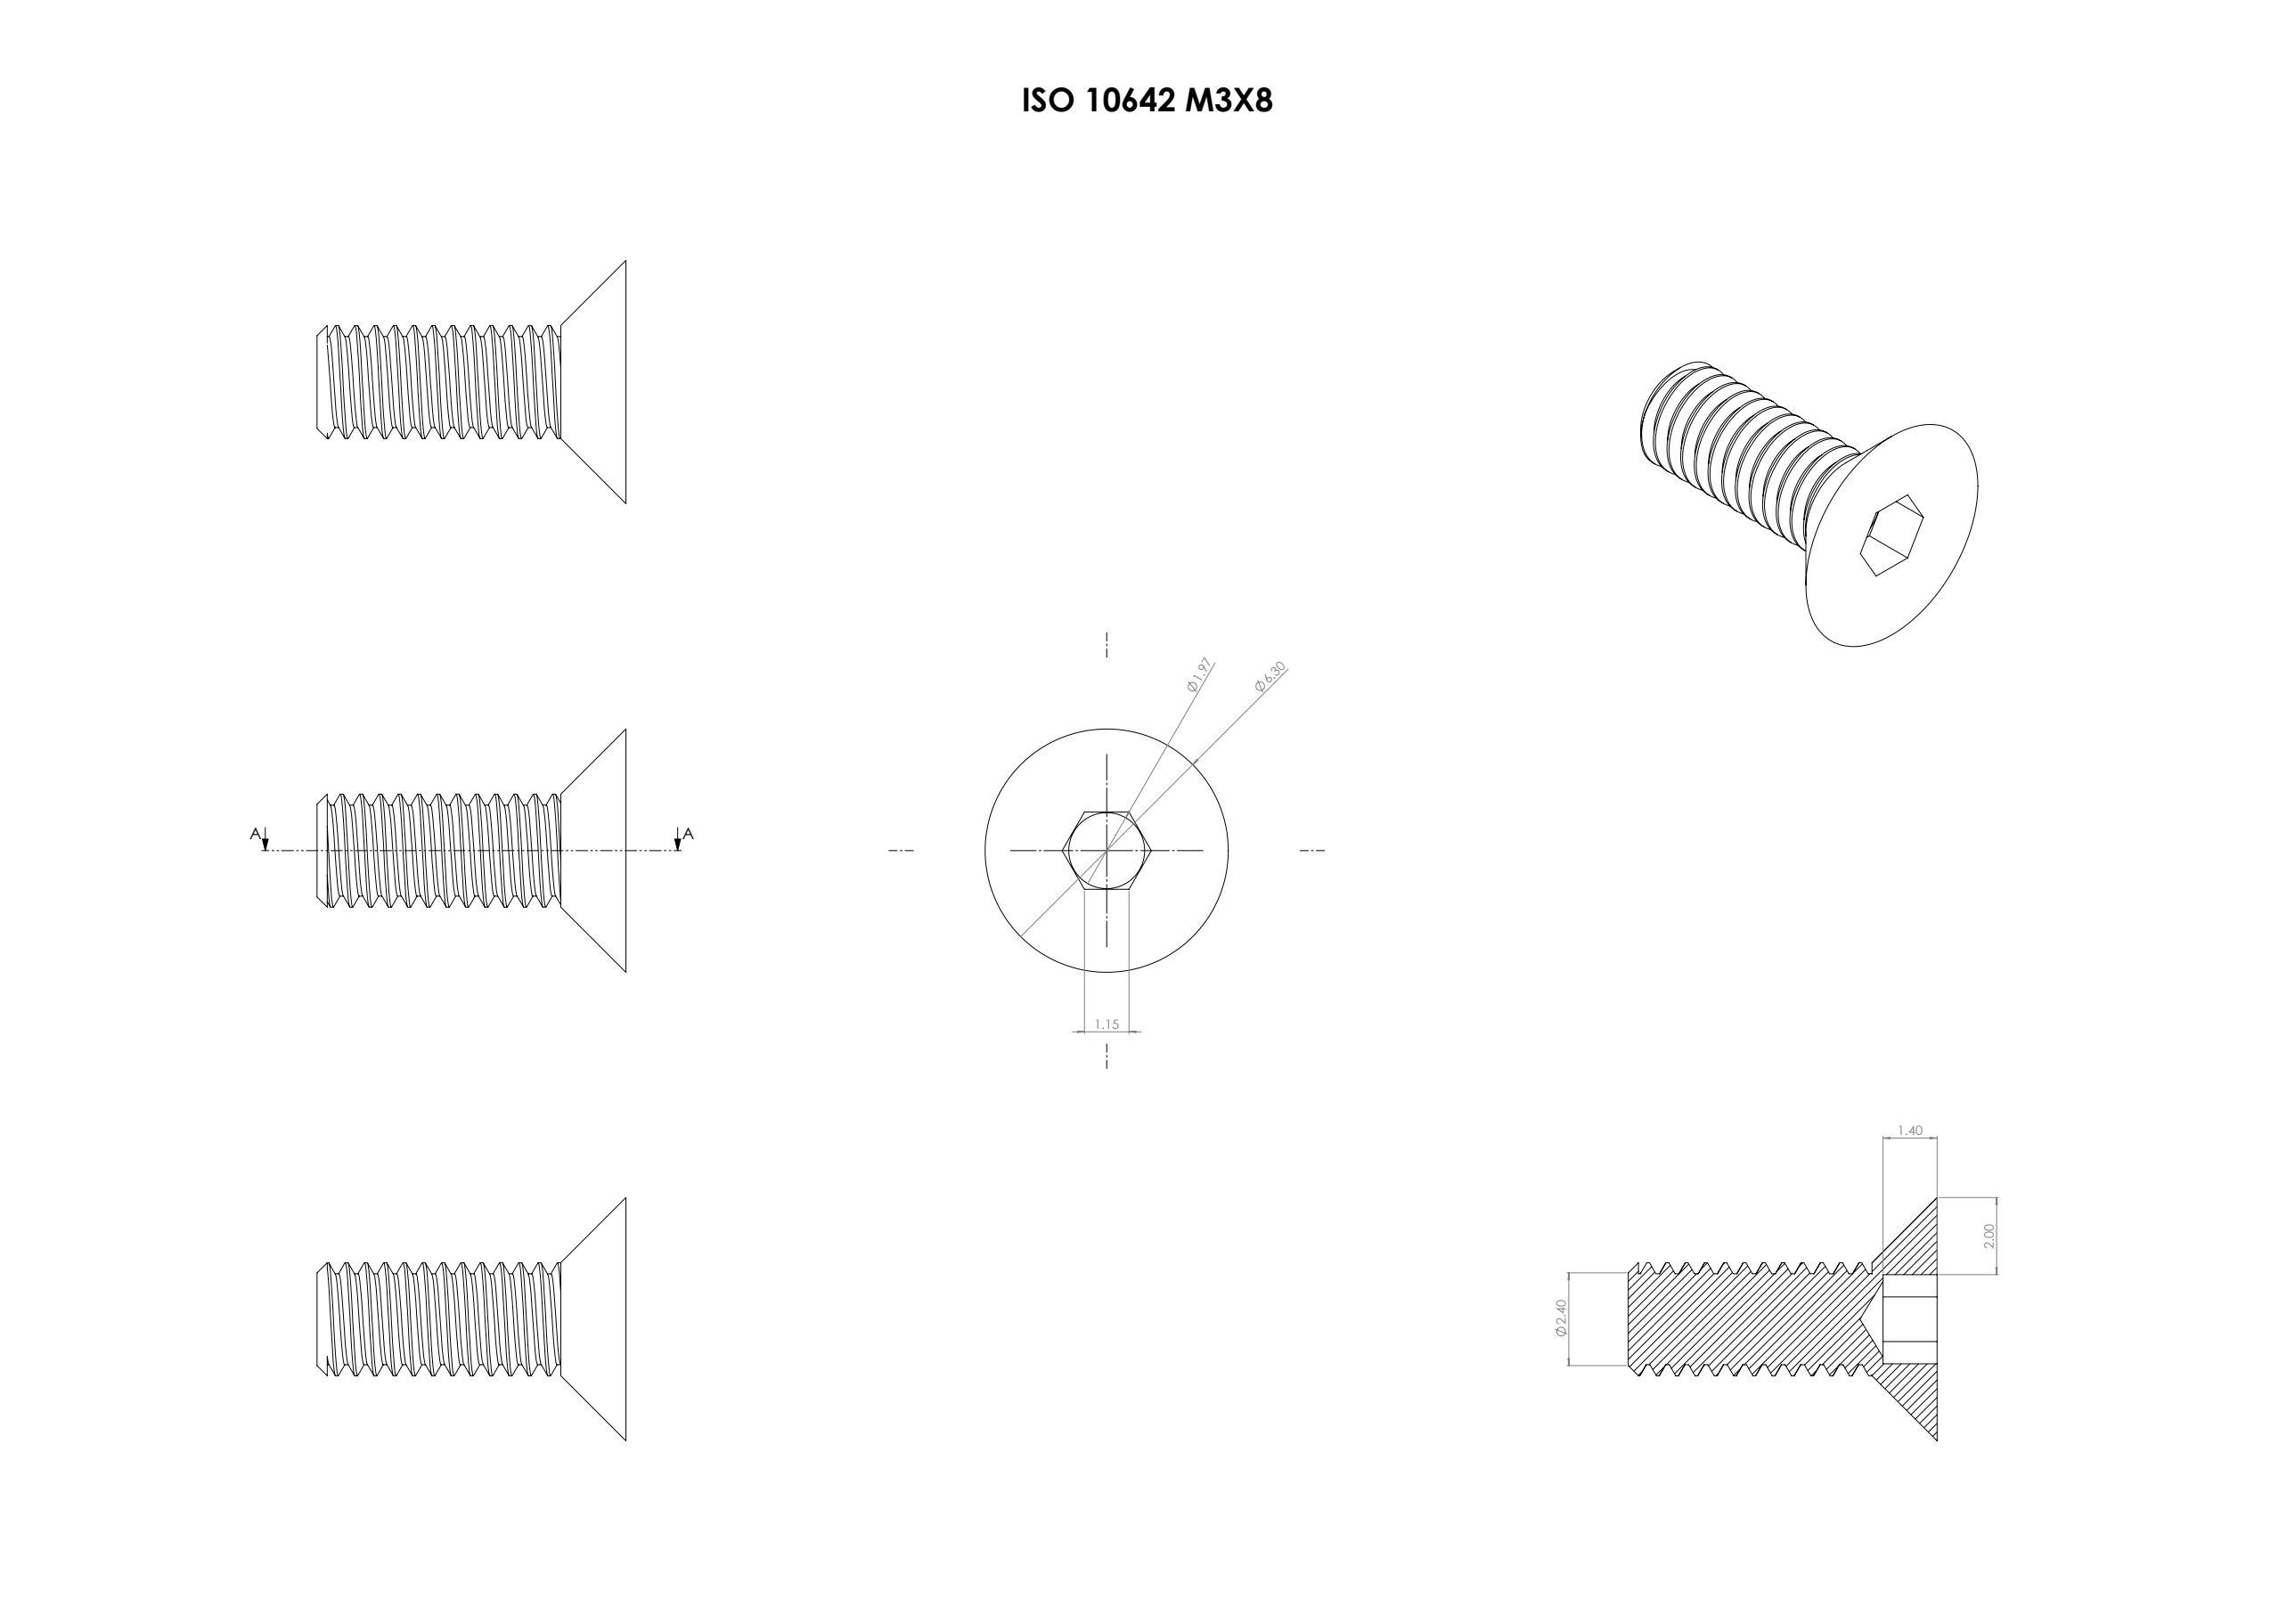
ISO-10303-21;
HEADER;
/* Generated by software containing ST-Developer
 * from STEP Tools, Inc. (www.steptools.com) 
 */

FILE_DESCRIPTION(
/* description */ (''),
/* implementation_level */ '2;1');

FILE_NAME(
/* name */ '11_ISO_10642_M3x8.step',
/* time_stamp */ '2026-10-21T01:59:45-07:00',
/* author */ (''),
/* organization */ (''),
/* preprocessor_version */ 'ST-DEVELOPER v20.2',
/* originating_system */ 'Autodesk Translation Framework v15.15.0.0',
/* authorisation */ '');

FILE_SCHEMA (('AUTOMOTIVE_DESIGN { 1 0 10303 214 3 1 1 }'));
ENDSEC;

DATA;
#10=MECHANICAL_DESIGN_GEOMETRIC_PRESENTATION_REPRESENTATION('',(#479),#18281);
#186=B_SPLINE_SURFACE_WITH_KNOTS('',3,3,((#17274,#17275,#17276,#17277,#17278,
#17279,#17280,#17281,#17282,#17283,#17284,#17285,#17286,#17287,#17288,#17289,
#17290,#17291,#17292,#17293,#17294,#17295,#17296,#17297,#17298,#17299,#17300,
#17301,#17302,#17303,#17304,#17305,#17306,#17307,#17308,#17309,#17310,#17311,
#17312,#17313,#17314,#17315,#17316,#17317,#17318,#17319,#17320,#17321,#17322,
#17323,#17324,#17325,#17326,#17327,#17328,#17329,#17330,#17331,#17332,#17333,
#17334,#17335,#17336,#17337,#17338,#17339,#17340,#17341,#17342,#17343,#17344,
#17345,#17346,#17347,#17348,#17349,#17350,#17351,#17352,#17353,#17354,#17355),
(#17356,#17357,#17358,#17359,#17360,#17361,#17362,#17363,#17364,#17365,
#17366,#17367,#17368,#17369,#17370,#17371,#17372,#17373,#17374,#17375,#17376,
#17377,#17378,#17379,#17380,#17381,#17382,#17383,#17384,#17385,#17386,#17387,
#17388,#17389,#17390,#17391,#17392,#17393,#17394,#17395,#17396,#17397,#17398,
#17399,#17400,#17401,#17402,#17403,#17404,#17405,#17406,#17407,#17408,#17409,
#17410,#17411,#17412,#17413,#17414,#17415,#17416,#17417,#17418,#17419,#17420,
#17421,#17422,#17423,#17424,#17425,#17426,#17427,#17428,#17429,#17430,#17431,
#17432,#17433,#17434,#17435,#17436,#17437),(#17438,#17439,#17440,#17441,
#17442,#17443,#17444,#17445,#17446,#17447,#17448,#17449,#17450,#17451,#17452,
#17453,#17454,#17455,#17456,#17457,#17458,#17459,#17460,#17461,#17462,#17463,
#17464,#17465,#17466,#17467,#17468,#17469,#17470,#17471,#17472,#17473,#17474,
#17475,#17476,#17477,#17478,#17479,#17480,#17481,#17482,#17483,#17484,#17485,
#17486,#17487,#17488,#17489,#17490,#17491,#17492,#17493,#17494,#17495,#17496,
#17497,#17498,#17499,#17500,#17501,#17502,#17503,#17504,#17505,#17506,#17507,
#17508,#17509,#17510,#17511,#17512,#17513,#17514,#17515,#17516,#17517,#17518,
#17519),(#17520,#17521,#17522,#17523,#17524,#17525,#17526,#17527,#17528,
#17529,#17530,#17531,#17532,#17533,#17534,#17535,#17536,#17537,#17538,#17539,
#17540,#17541,#17542,#17543,#17544,#17545,#17546,#17547,#17548,#17549,#17550,
#17551,#17552,#17553,#17554,#17555,#17556,#17557,#17558,#17559,#17560,#17561,
#17562,#17563,#17564,#17565,#17566,#17567,#17568,#17569,#17570,#17571,#17572,
#17573,#17574,#17575,#17576,#17577,#17578,#17579,#17580,#17581,#17582,#17583,
#17584,#17585,#17586,#17587,#17588,#17589,#17590,#17591,#17592,#17593,#17594,
#17595,#17596,#17597,#17598,#17599,#17600,#17601)),.UNSPECIFIED.,.F.,.F.,
 .F.,(4,4),(4,1,1,1,1,1,1,1,1,1,1,1,1,1,1,1,1,1,1,1,1,1,1,1,1,1,1,1,1,1,
1,1,1,1,1,1,1,1,1,1,1,1,1,1,1,1,1,1,1,1,1,1,1,1,1,1,1,1,1,1,1,1,1,1,1,1,
1,1,1,1,1,1,1,1,1,1,1,1,1,4),(0.,0.0329955678841871),(8.30203615430834,
9.29064014026014,10.2792441262119,11.2678481121638,12.2564520981156,13.2450560840674,
14.2336600700192,15.222264055971,16.2108680419228,17.1994720278746,18.1880760138264,
19.1766799997782,20.16528398573,21.1538879716818,22.1424919576336,23.1310959435854,
24.1196999295372,25.108303915489,26.0969079014409,27.0855118873927,28.0741158733445,
29.0627198592963,30.0513238452481,31.0399278311999,32.0285318171517,33.0171358031035,
34.0057397890553,34.9943437750071,35.9829477609589,36.9715517469107,37.9601557328625,
38.9487597188143,39.9373637047661,40.9259676907179,41.9145716766698,42.9031756626216,
43.8917796485734,44.8803836345252,45.868987620477,46.8575916064288,47.8461955923806,
48.8347995783324,49.8234035642842,50.812007550236,51.8006115361878,52.7892155221396,
53.7778195080914,54.7664234940432,55.755027479995,56.7436314659468,57.7322354518986,
58.7208394378505,59.7094434238023,60.6980474097541,61.6866513957059,62.6752553816577,
63.6638593676095,64.6524633535613,65.6410673395131,66.6296713254649,67.6182753114167,
68.6068792973685,69.5954832833203,70.5840872692721,71.5726912552239,72.5612952411758,
73.5498992271276,74.5385032130794,75.5271071990312,76.515711184983,77.5043151709348,
78.4929191568866,79.4815231428384,80.4701271287902,81.458731114742,82.4473351006938,
83.4359390866456,84.4245430725974,85.4131470585492,86.401751044501),
 .UNSPECIFIED.);
#187=B_SPLINE_SURFACE_WITH_KNOTS('',3,3,((#17813,#17814,#17815,#17816,#17817,
#17818,#17819,#17820,#17821,#17822,#17823,#17824,#17825,#17826,#17827,#17828,
#17829,#17830,#17831,#17832,#17833,#17834,#17835,#17836,#17837,#17838,#17839,
#17840,#17841,#17842,#17843,#17844,#17845,#17846,#17847,#17848,#17849,#17850,
#17851,#17852,#17853,#17854,#17855,#17856,#17857,#17858,#17859,#17860,#17861,
#17862,#17863,#17864,#17865,#17866,#17867,#17868,#17869,#17870,#17871,#17872,
#17873,#17874,#17875,#17876,#17877,#17878,#17879,#17880,#17881,#17882,#17883,
#17884,#17885,#17886,#17887,#17888,#17889,#17890,#17891,#17892,#17893,#17894),
(#17895,#17896,#17897,#17898,#17899,#17900,#17901,#17902,#17903,#17904,
#17905,#17906,#17907,#17908,#17909,#17910,#17911,#17912,#17913,#17914,#17915,
#17916,#17917,#17918,#17919,#17920,#17921,#17922,#17923,#17924,#17925,#17926,
#17927,#17928,#17929,#17930,#17931,#17932,#17933,#17934,#17935,#17936,#17937,
#17938,#17939,#17940,#17941,#17942,#17943,#17944,#17945,#17946,#17947,#17948,
#17949,#17950,#17951,#17952,#17953,#17954,#17955,#17956,#17957,#17958,#17959,
#17960,#17961,#17962,#17963,#17964,#17965,#17966,#17967,#17968,#17969,#17970,
#17971,#17972,#17973,#17974,#17975,#17976),(#17977,#17978,#17979,#17980,
#17981,#17982,#17983,#17984,#17985,#17986,#17987,#17988,#17989,#17990,#17991,
#17992,#17993,#17994,#17995,#17996,#17997,#17998,#17999,#18000,#18001,#18002,
#18003,#18004,#18005,#18006,#18007,#18008,#18009,#18010,#18011,#18012,#18013,
#18014,#18015,#18016,#18017,#18018,#18019,#18020,#18021,#18022,#18023,#18024,
#18025,#18026,#18027,#18028,#18029,#18030,#18031,#18032,#18033,#18034,#18035,
#18036,#18037,#18038,#18039,#18040,#18041,#18042,#18043,#18044,#18045,#18046,
#18047,#18048,#18049,#18050,#18051,#18052,#18053,#18054,#18055,#18056,#18057,
#18058),(#18059,#18060,#18061,#18062,#18063,#18064,#18065,#18066,#18067,
#18068,#18069,#18070,#18071,#18072,#18073,#18074,#18075,#18076,#18077,#18078,
#18079,#18080,#18081,#18082,#18083,#18084,#18085,#18086,#18087,#18088,#18089,
#18090,#18091,#18092,#18093,#18094,#18095,#18096,#18097,#18098,#18099,#18100,
#18101,#18102,#18103,#18104,#18105,#18106,#18107,#18108,#18109,#18110,#18111,
#18112,#18113,#18114,#18115,#18116,#18117,#18118,#18119,#18120,#18121,#18122,
#18123,#18124,#18125,#18126,#18127,#18128,#18129,#18130,#18131,#18132,#18133,
#18134,#18135,#18136,#18137,#18138,#18139,#18140)),.UNSPECIFIED.,.F.,.F.,
 .F.,(4,4),(4,1,1,1,1,1,1,1,1,1,1,1,1,1,1,1,1,1,1,1,1,1,1,1,1,1,1,1,1,1,
1,1,1,1,1,1,1,1,1,1,1,1,1,1,1,1,1,1,1,1,1,1,1,1,1,1,1,1,1,1,1,1,1,1,1,1,
1,1,1,1,1,1,1,1,1,1,1,1,1,4),(0.,0.0329955678841871),(11.6159397475004,
12.6045437334522,13.593147719404,14.5817517053558,15.5703556913076,16.5589596772594,
17.5475636632112,18.536167649163,19.5247716351148,20.5133756210666,21.5019796070184,
22.4905835929702,23.479187578922,24.4677915648739,25.4563955508257,26.4449995367775,
27.4336035227293,28.4222075086811,29.4108114946329,30.3994154805847,31.3880194665365,
32.3766234524883,33.3652274384401,34.3538314243919,35.3424354103437,36.3310393962955,
37.3196433822473,38.3082473681991,39.296851354151,40.2854553401028,41.2740593260546,
42.2626633120064,43.2512672979582,44.23987128391,45.2284752698618,46.2170792558136,
47.2056832417654,48.1942872277172,49.182891213669,50.1714951996208,51.1600991855726,
52.1487031715244,53.1373071574762,54.1259111434281,55.1145151293799,56.1031191153317,
57.0917231012835,58.0803270872353,59.0689310731871,60.0575350591389,61.0461390450907,
62.0347430310425,63.0233470169943,64.0119510029461,65.0005549888979,65.9891589748497,
66.9777629608015,67.9663669467533,68.9549709327052,69.943574918657,70.9321789046088,
71.9207828905606,72.9093868765124,73.8979908624642,74.886594848416,75.8751988343678,
76.8638028203196,77.8524068062714,78.8410107922232,79.829614778175,80.8182187641268,
81.8068227500786,82.7954267360304,83.7840307219822,84.7726347079341,85.7612386938859,
86.7498426798377,87.7384466657895,88.7270506517413,89.7156546376931),
 .UNSPECIFIED.);
#312=B_SPLINE_CURVE_WITH_KNOTS('',3,(#16240,#16241,#16242,#16243,#16244,
#16245,#16246,#16247,#16248,#16249),.UNSPECIFIED.,.F.,.F.,(4,3,3,4),(-4.09202352044854,
-3.95441594380723,-2.96581195785542,-2.07317267331972),.UNSPECIFIED.);
#313=B_SPLINE_CURVE_WITH_KNOTS('',3,(#16252,#16253,#16254,#16255,#16256,
#16257,#16258),.UNSPECIFIED.,.F.,.F.,(4,3,4),(0.,0.98860398595181,1.12274180646091),
 .UNSPECIFIED.);
#314=B_SPLINE_CURVE_WITH_KNOTS('',3,(#16263,#16264,#16265,#16266,#16267,
#16268,#16269,#16270,#16271,#16272,#16273,#16274,#16275,#16276,#16277,#16278,
#16279,#16280,#16281,#16282,#16283,#16284),.UNSPECIFIED.,.F.,.F.,(4,3,3,
3,3,3,3,4),(-10.3752088276281,-9.88603985951807,-8.89743587356626,-7.90883188761445,
-6.92022790166265,-5.93162391571084,-4.94301992975903,-4.09202352044854),
 .UNSPECIFIED.);
#315=B_SPLINE_CURVE_WITH_KNOTS('',3,(#16285,#16286,#16287,#16288,#16289,
#16290,#16291,#16292,#16293,#16294,#16295,#16296,#16297,#16298,#16299,#16300,
#16301,#16302,#16303,#16304,#16305,#16306),.UNSPECIFIED.,.F.,.F.,(4,3,3,
3,3,3,3,4),(1.12274180646091,1.97720797190362,2.96581195785542,3.95441594380723,
4.94301992975904,5.93162391571084,6.92022790166265,7.4059271136405),
 .UNSPECIFIED.);
#316=B_SPLINE_CURVE_WITH_KNOTS('',3,(#16311,#16312,#16313,#16314,#16315,
#16316,#16317,#16318,#16319,#16320,#16321,#16322,#16323,#16324,#16325,#16326,
#16327,#16328,#16329,#16330,#16331,#16332),.UNSPECIFIED.,.F.,.F.,(4,3,3,
3,3,3,3,4),(-16.6583941348077,-15.8176637752289,-14.8290597892771,-13.8404558033253,
-12.8518518173735,-11.8632478314217,-10.8746438454699,-10.3752088276281),
 .UNSPECIFIED.);
#317=B_SPLINE_CURVE_WITH_KNOTS('',3,(#16333,#16334,#16335,#16336,#16337,
#16338,#16339,#16340,#16341,#16342,#16343,#16344,#16345,#16346,#16347,#16348,
#16349,#16350,#16351,#16352,#16353,#16354),.UNSPECIFIED.,.F.,.F.,(4,3,3,
3,3,3,3,4),(7.4059271136405,7.90883188761445,8.89743587356626,9.88603985951806,
10.8746438454699,11.8632478314217,12.8518518173735,13.6891124208201),
 .UNSPECIFIED.);
#318=B_SPLINE_CURVE_WITH_KNOTS('',3,(#16359,#16360,#16361,#16362,#16363,
#16364,#16365,#16366,#16367,#16368,#16369,#16370,#16371,#16372,#16373,#16374,
#16375,#16376,#16377,#16378,#16379,#16380,#16381,#16382,#16383),
 .UNSPECIFIED.,.F.,.F.,(4,3,3,3,3,3,3,3,4),(-22.9415794419873,-22.7378916768916,
-21.7492876909397,-20.7606837049879,-19.7720797190361,-18.7834757330843,
-17.7948717471325,-16.8062677611807,-16.6583941348077),.UNSPECIFIED.);
#319=B_SPLINE_CURVE_WITH_KNOTS('',3,(#16384,#16385,#16386,#16387,#16388,
#16389,#16390,#16391,#16392,#16393,#16394,#16395,#16396,#16397,#16398,#16399,
#16400,#16401,#16402,#16403,#16404,#16405,#16406,#16407,#16408),
 .UNSPECIFIED.,.F.,.F.,(4,3,3,3,3,3,3,3,4),(13.6891124208201,13.8404558033253,
14.8290597892771,15.8176637752289,16.8062677611807,17.7948717471325,18.7834757330843,
19.7720797190361,19.9722977279997),.UNSPECIFIED.);
#320=B_SPLINE_CURVE_WITH_KNOTS('',3,(#16413,#16414,#16415,#16416,#16417,
#16418,#16419,#16420,#16421,#16422,#16423,#16424,#16425,#16426,#16427,#16428,
#16429,#16430,#16431,#16432,#16433,#16434),.UNSPECIFIED.,.F.,.F.,(4,3,3,
3,3,3,3,4),(-29.2247647491669,-28.6695155926024,-27.6809116066506,-26.6923076206988,
-25.703703634747,-24.7150996487952,-23.7264956628434,-22.9415794419873),
 .UNSPECIFIED.);
#321=B_SPLINE_CURVE_WITH_KNOTS('',3,(#16435,#16436,#16437,#16438,#16439,
#16440,#16441,#16442,#16443,#16444,#16445,#16446,#16447,#16448,#16449,#16450,
#16451,#16452,#16453,#16454,#16455,#16456),.UNSPECIFIED.,.F.,.F.,(4,3,3,
3,3,3,3,4),(19.9722977279997,20.7606837049879,21.7492876909397,22.7378916768916,
23.7264956628434,24.7150996487952,25.703703634747,26.2554830351793),
 .UNSPECIFIED.);
#322=B_SPLINE_CURVE_WITH_KNOTS('',3,(#16461,#16462,#16463,#16464,#16465,
#16466,#16467,#16468,#16469,#16470,#16471,#16472,#16473,#16474,#16475,#16476,
#16477,#16478,#16479,#16480,#16481,#16482),.UNSPECIFIED.,.F.,.F.,(4,3,3,
3,3,3,3,4),(-35.5079500563465,-34.6011395083132,-33.6125355223614,-32.6239315364096,
-31.6353275504578,-30.646723564506,-29.6581195785542,-29.2247647491669),
 .UNSPECIFIED.);
#323=B_SPLINE_CURVE_WITH_KNOTS('',3,(#16483,#16484,#16485,#16486,#16487,
#16488,#16489,#16490,#16491,#16492,#16493,#16494,#16495,#16496,#16497,#16498,
#16499,#16500,#16501,#16502,#16503,#16504),.UNSPECIFIED.,.F.,.F.,(4,3,3,
3,3,3,3,4),(26.2554830351793,26.6923076206988,27.6809116066506,28.6695155926024,
29.6581195785542,30.646723564506,31.6353275504578,32.5386683423588),
 .UNSPECIFIED.);
#324=B_SPLINE_CURVE_WITH_KNOTS('',3,(#16509,#16510,#16511,#16512,#16513,
#16514,#16515,#16516,#16517,#16518,#16519,#16520,#16521,#16522,#16523,#16524,
#16525,#16526,#16527,#16528,#16529,#16530,#16531,#16532,#16533),
 .UNSPECIFIED.,.F.,.F.,(4,3,3,3,3,3,3,3,4),(-41.7911353635261,-41.5213674099759,
-40.5327634240241,-39.5441594380723,-38.5555554521205,-37.5669514661687,
-36.5783474802168,-35.589743494265,-35.5079500563465),.UNSPECIFIED.);
#325=B_SPLINE_CURVE_WITH_KNOTS('',3,(#16534,#16535,#16536,#16537,#16538,
#16539,#16540,#16541,#16542,#16543,#16544,#16545,#16546,#16547,#16548,#16549,
#16550,#16551,#16552,#16553,#16554,#16555,#16556,#16557,#16558),
 .UNSPECIFIED.,.F.,.F.,(4,3,3,3,3,3,3,3,4),(32.5386683423588,32.6239315364096,
33.6125355223614,34.6011395083132,35.589743494265,36.5783474802168,37.5669514661686,
38.5555554521205,38.8218536495384),.UNSPECIFIED.);
#326=B_SPLINE_CURVE_WITH_KNOTS('',3,(#16563,#16564,#16565,#16566,#16567,
#16568,#16569,#16570,#16571,#16572,#16573,#16574,#16575,#16576,#16577,#16578,
#16579,#16580,#16581,#16582,#16583,#16584),.UNSPECIFIED.,.F.,.F.,(4,3,3,
3,3,3,3,4),(-48.0743206707057,-47.4529913256867,-46.4643873397349,-45.4757833537831,
-44.4871793678313,-43.4985753818795,-42.5099713959277,-41.7911353635261),
 .UNSPECIFIED.);
#327=B_SPLINE_CURVE_WITH_KNOTS('',3,(#16585,#16586,#16587,#16588,#16589,
#16590,#16591,#16592,#16593,#16594,#16595,#16596,#16597,#16598,#16599,#16600,
#16601,#16602,#16603,#16604,#16605,#16606),.UNSPECIFIED.,.F.,.F.,(4,3,3,
3,3,3,3,4),(38.8218536495384,39.5441594380723,40.5327634240241,41.5213674099759,
42.5099713959277,43.4985753818795,44.4871793678313,45.105038956718),
 .UNSPECIFIED.);
#328=B_SPLINE_CURVE_WITH_KNOTS('',3,(#16611,#16612,#16613,#16614,#16615,
#16616,#16617,#16618,#16619,#16620,#16621,#16622,#16623,#16624,#16625,#16626,
#16627,#16628,#16629,#16630,#16631,#16632),.UNSPECIFIED.,.F.,.F.,(4,3,3,
3,3,3,3,4),(-54.3575059778853,-53.3846152413976,-52.3960112554458,-51.4074072694939,
-50.4188032835421,-49.4301992975903,-48.4415953116385,-48.0743206707057),
 .UNSPECIFIED.);
#329=B_SPLINE_CURVE_WITH_KNOTS('',3,(#16633,#16634,#16635,#16636,#16637,
#16638,#16639,#16640,#16641,#16642,#16643,#16644,#16645,#16646,#16647,#16648,
#16649,#16650,#16651,#16652,#16653,#16654),.UNSPECIFIED.,.F.,.F.,(4,3,3,
3,3,3,3,4),(45.105038956718,45.4757833537831,46.4643873397349,47.4529913256867,
48.4415953116385,49.4301992975903,50.4188032835421,51.3882242638976),
 .UNSPECIFIED.);
#330=B_SPLINE_CURVE_WITH_KNOTS('',3,(#16659,#16660,#16661,#16662,#16663,
#16664,#16665,#16666,#16667,#16668,#16669,#16670,#16671,#16672,#16673,#16674,
#16675,#16676,#16677,#16678,#16679,#16680,#16681,#16682,#16683),
 .UNSPECIFIED.,.F.,.F.,(4,3,3,3,3,3,3,3,4),(-60.6406912850648,-60.3048431430602,
-59.3162391571084,-58.3276351711566,-57.3390311852048,-56.350427199253,
-55.3618232133012,-54.3732192273494,-54.3575059778853),.UNSPECIFIED.);
#331=B_SPLINE_CURVE_WITH_KNOTS('',3,(#16684,#16685,#16686,#16687,#16688,
#16689,#16690,#16691,#16692,#16693,#16694,#16695,#16696,#16697,#16698,#16699,
#16700,#16701,#16702,#16703,#16704,#16705,#16706,#16707,#16708),
 .UNSPECIFIED.,.F.,.F.,(4,3,3,3,3,3,3,3,4),(51.3882242638976,51.4074072694939,
52.3960112554457,53.3846152413976,54.3732192273494,55.3618232133012,56.350427199253,
57.3390311852048,57.6714095710772),.UNSPECIFIED.);
#332=B_SPLINE_CURVE_WITH_KNOTS('',3,(#16713,#16714,#16715,#16716,#16717,
#16718,#16719,#16720,#16721,#16722,#16723,#16724,#16725,#16726,#16727,#16728,
#16729,#16730,#16731,#16732,#16733,#16734),.UNSPECIFIED.,.F.,.F.,(4,3,3,
3,3,3,3,4),(-66.9238765922444,-66.236467058771,-65.2478630728192,-64.2592590868674,
-63.2706551009156,-62.2820511149638,-61.293447129012,-60.6406912850648),
 .UNSPECIFIED.);
#333=B_SPLINE_CURVE_WITH_KNOTS('',3,(#16735,#16736,#16737,#16738,#16739,
#16740,#16741,#16742,#16743,#16744,#16745,#16746,#16747,#16748,#16749,#16750,
#16751,#16752,#16753,#16754,#16755,#16756),.UNSPECIFIED.,.F.,.F.,(4,3,3,
3,3,3,3,4),(57.6714095710772,58.3276351711566,59.3162391571084,60.3048431430602,
61.293447129012,62.2820511149638,63.2706551009156,63.9545948782568),
 .UNSPECIFIED.);
#334=B_SPLINE_CURVE_WITH_KNOTS('',3,(#16761,#16762,#16763,#16764,#16765,
#16766,#16767,#16768,#16769,#16770,#16771,#16772,#16773,#16774,#16775,#16776,
#16777,#16778,#16779,#16780,#16781,#16782,#16783,#16784,#16785),
 .UNSPECIFIED.,.F.,.F.,(4,3,3,3,3,3,3,3,4),(-73.207061899424,-73.1566949604337,
-72.1680909744819,-71.1794869885301,-70.1908830025783,-69.2022790166264,
-68.2136750306747,-67.2250710447229,-66.9238765922444),.UNSPECIFIED.);
#335=B_SPLINE_CURVE_WITH_KNOTS('',3,(#16786,#16787,#16788,#16789,#16790,
#16791,#16792,#16793,#16794,#16795,#16796,#16797,#16798,#16799,#16800,#16801,
#16802,#16803,#16804,#16805,#16806,#16807,#16808,#16809,#16810),
 .UNSPECIFIED.,.F.,.F.,(4,3,3,3,3,3,3,3,4),(63.9545948782568,64.2592590868674,
65.2478630728192,66.236467058771,67.2250710447228,68.2136750306746,69.2022790166264,
70.1908830025782,70.2377801854364),.UNSPECIFIED.);
#336=B_SPLINE_CURVE_WITH_KNOTS('',3,(#16816,#16817,#16818,#16819,#16820,
#16821),.UNSPECIFIED.,.F.,.F.,(4,1,1,4),(84.8230016469244,85.7612386938859,
86.7498426798377,87.6424819643734),.UNSPECIFIED.);
#337=B_SPLINE_CURVE_WITH_KNOTS('',3,(#16824,#16825,#16826,#16827,#16828),
 .UNSPECIFIED.,.F.,.F.,(4,1,4),(84.8230016469244,85.4131470585492,86.401751044501),
 .UNSPECIFIED.);
#338=B_SPLINE_CURVE_WITH_KNOTS('',3,(#16833,#16834,#16835,#16836,#16837,
#16838,#16839,#16840,#16841,#16842,#16843),.UNSPECIFIED.,.F.,.F.,(4,1,1,
1,1,1,1,1,4),(78.5398163397448,78.8410107922232,79.829614778175,80.8182187641268,
81.8068227500786,82.7954267360304,83.7840307219822,84.7726347079341,84.8230016469244),
 .UNSPECIFIED.);
#339=B_SPLINE_CURVE_WITH_KNOTS('',3,(#16844,#16845,#16846,#16847,#16848,
#16849,#16850,#16851,#16852,#16853),.UNSPECIFIED.,.F.,.F.,(4,1,1,1,1,1,
1,4),(78.5398163397448,79.4815231428384,80.4701271287902,81.458731114742,
82.4473351006938,83.4359390866456,84.4245430725974,84.8230016469244),
 .UNSPECIFIED.);
#340=B_SPLINE_CURVE_WITH_KNOTS('',3,(#16858,#16859,#16860,#16861,#16862,
#16863,#16864,#16865,#16866,#16867),.UNSPECIFIED.,.F.,.F.,(4,1,1,1,1,1,
1,4),(72.2566310325652,72.9093868765124,73.8979908624642,74.886594848416,
75.8751988343678,76.8638028203196,77.8524068062714,78.5398163397448),
 .UNSPECIFIED.);
#341=B_SPLINE_CURVE_WITH_KNOTS('',3,(#16868,#16869,#16870,#16871,#16872,
#16873,#16874,#16875,#16876,#16877,#16878),.UNSPECIFIED.,.F.,.F.,(4,1,1,
1,1,1,1,1,4),(72.2566310325652,72.5612952411758,73.5498992271276,74.5385032130794,
75.5271071990312,76.515711184983,77.5043151709348,78.4929191568866,78.5398163397448),
 .UNSPECIFIED.);
#342=B_SPLINE_CURVE_WITH_KNOTS('',3,(#16883,#16884,#16885,#16886,#16887,
#16888,#16889,#16890,#16891,#16892,#16893),.UNSPECIFIED.,.F.,.F.,(4,1,1,
1,1,1,1,1,4),(65.9734457253856,65.9891589748497,66.9777629608015,67.9663669467533,
68.9549709327052,69.943574918657,70.9321789046088,71.9207828905606,72.2566310325652),
 .UNSPECIFIED.);
#343=B_SPLINE_CURVE_WITH_KNOTS('',3,(#16894,#16895,#16896,#16897,#16898,
#16899,#16900,#16901,#16902,#16903),.UNSPECIFIED.,.F.,.F.,(4,1,1,1,1,1,
1,4),(65.9734457253856,66.6296713254649,67.6182753114167,68.6068792973685,
69.5954832833203,70.5840872692721,71.5726912552239,72.2566310325652),
 .UNSPECIFIED.);
#344=B_SPLINE_CURVE_WITH_KNOTS('',3,(#16908,#16909,#16910,#16911,#16912,
#16913,#16914,#16915,#16916,#16917),.UNSPECIFIED.,.F.,.F.,(4,1,1,1,1,1,
1,4),(59.6902604182061,60.0575350591389,61.0461390450907,62.0347430310425,
63.0233470169943,64.0119510029461,65.0005549888979,65.9734457253856),
 .UNSPECIFIED.);
#345=B_SPLINE_CURVE_WITH_KNOTS('',3,(#16918,#16919,#16920,#16921,#16922,
#16923,#16924,#16925,#16926,#16927,#16928),.UNSPECIFIED.,.F.,.F.,(4,1,1,
1,1,1,1,1,4),(59.690260418206,59.7094434238023,60.6980474097541,61.6866513957059,
62.6752553816577,63.6638593676095,64.6524633535613,65.6410673395131,65.9734457253856),
 .UNSPECIFIED.);
#346=B_SPLINE_CURVE_WITH_KNOTS('',3,(#16933,#16934,#16935,#16936,#16937,
#16938,#16939,#16940,#16941,#16942),.UNSPECIFIED.,.F.,.F.,(4,1,1,1,1,1,
1,4),(53.4070751110265,54.1259111434281,55.1145151293799,56.1031191153317,
57.0917231012835,58.0803270872353,59.0689310731871,59.6902604182061),
 .UNSPECIFIED.);
#347=B_SPLINE_CURVE_WITH_KNOTS('',3,(#16943,#16944,#16945,#16946,#16947,
#16948,#16949,#16950,#16951,#16952),.UNSPECIFIED.,.F.,.F.,(4,1,1,1,1,1,
1,4),(53.4070751110264,53.7778195080914,54.7664234940432,55.755027479995,
56.7436314659468,57.7322354518986,58.7208394378505,59.690260418206),
 .UNSPECIFIED.);
#348=B_SPLINE_CURVE_WITH_KNOTS('',3,(#16957,#16958,#16959,#16960,#16961,
#16962,#16963,#16964,#16965,#16966,#16967),.UNSPECIFIED.,.F.,.F.,(4,1,1,
1,1,1,1,1,4),(47.1238898038469,47.2056832417654,48.1942872277172,49.182891213669,
50.1714951996208,51.1600991855726,52.1487031715244,53.1373071574762,53.4070751110265),
 .UNSPECIFIED.);
#349=B_SPLINE_CURVE_WITH_KNOTS('',3,(#16968,#16969,#16970,#16971,#16972,
#16973,#16974,#16975,#16976,#16977),.UNSPECIFIED.,.F.,.F.,(4,1,1,1,1,1,
1,4),(47.1238898038468,47.8461955923806,48.8347995783324,49.8234035642842,
50.812007550236,51.8006115361878,52.7892155221396,53.4070751110264),
 .UNSPECIFIED.);
#350=B_SPLINE_CURVE_WITH_KNOTS('',3,(#16982,#16983,#16984,#16985,#16986,
#16987,#16988,#16989,#16990,#16991),.UNSPECIFIED.,.F.,.F.,(4,1,1,1,1,1,
1,4),(40.8407044966673,41.2740593260546,42.2626633120064,43.2512672979582,
44.23987128391,45.2284752698618,46.2170792558136,47.1238898038469),
 .UNSPECIFIED.);
#351=B_SPLINE_CURVE_WITH_KNOTS('',3,(#16992,#16993,#16994,#16995,#16996,
#16997,#16998,#16999,#17000,#17001,#17002),.UNSPECIFIED.,.F.,.F.,(4,1,1,
1,1,1,1,1,4),(40.8407044966673,40.9259676907179,41.9145716766698,42.9031756626216,
43.8917796485734,44.8803836345252,45.868987620477,46.8575916064288,47.1238898038468),
 .UNSPECIFIED.);
#352=B_SPLINE_CURVE_WITH_KNOTS('',3,(#17007,#17008,#17009,#17010,#17011,
#17012,#17013,#17014,#17015,#17016),.UNSPECIFIED.,.F.,.F.,(4,1,1,1,1,1,
1,4),(34.5575191894877,35.3424354103437,36.3310393962955,37.3196433822473,
38.3082473681991,39.296851354151,40.2854553401028,40.8407044966673),
 .UNSPECIFIED.);
#353=B_SPLINE_CURVE_WITH_KNOTS('',3,(#17017,#17018,#17019,#17020,#17021,
#17022,#17023,#17024,#17025,#17026),.UNSPECIFIED.,.F.,.F.,(4,1,1,1,1,1,
1,4),(34.5575191894877,34.9943437750071,35.9829477609589,36.9715517469107,
37.9601557328625,38.9487597188143,39.9373637047661,40.8407044966673),
 .UNSPECIFIED.);
#354=B_SPLINE_CURVE_WITH_KNOTS('',3,(#17031,#17032,#17033,#17034,#17035,
#17036,#17037,#17038,#17039,#17040,#17041),.UNSPECIFIED.,.F.,.F.,(4,1,1,
1,1,1,1,1,4),(28.2743338823081,28.4222075086811,29.4108114946329,30.3994154805847,
31.3880194665365,32.3766234524883,33.3652274384401,34.3538314243919,34.5575191894877),
 .UNSPECIFIED.);
#355=B_SPLINE_CURVE_WITH_KNOTS('',3,(#17042,#17043,#17044,#17045,#17046,
#17047,#17048,#17049,#17050,#17051),.UNSPECIFIED.,.F.,.F.,(4,1,1,1,1,1,
1,4),(28.2743338823081,29.0627198592963,30.0513238452481,31.0399278311999,
32.0285318171517,33.0171358031035,34.0057397890553,34.5575191894877),
 .UNSPECIFIED.);
#356=B_SPLINE_CURVE_WITH_KNOTS('',3,(#17056,#17057,#17058,#17059,#17060,
#17061,#17062,#17063,#17064,#17065),.UNSPECIFIED.,.F.,.F.,(4,1,1,1,1,1,
1,4),(21.9911485751285,22.4905835929702,23.479187578922,24.4677915648739,
25.4563955508257,26.4449995367775,27.4336035227293,28.2743338823081),
 .UNSPECIFIED.);
#357=B_SPLINE_CURVE_WITH_KNOTS('',3,(#17066,#17067,#17068,#17069,#17070,
#17071,#17072,#17073,#17074,#17075,#17076),.UNSPECIFIED.,.F.,.F.,(4,1,1,
1,1,1,1,1,4),(21.9911485751285,22.1424919576336,23.1310959435854,24.1196999295372,
25.108303915489,26.0969079014409,27.0855118873927,28.0741158733445,28.2743338823081),
 .UNSPECIFIED.);
#358=B_SPLINE_CURVE_WITH_KNOTS('',3,(#17081,#17082,#17083,#17084,#17085,
#17086,#17087,#17088,#17089,#17090),.UNSPECIFIED.,.F.,.F.,(4,1,1,1,1,1,
1,4),(15.7079632679489,16.5589596772594,17.5475636632112,18.536167649163,
19.5247716351148,20.5133756210666,21.5019796070184,21.9911485751285),
 .UNSPECIFIED.);
#359=B_SPLINE_CURVE_WITH_KNOTS('',3,(#17091,#17092,#17093,#17094,#17095,
#17096,#17097,#17098,#17099,#17100),.UNSPECIFIED.,.F.,.F.,(4,1,1,1,1,1,
1,4),(15.7079632679489,16.2108680419228,17.1994720278746,18.1880760138264,
19.1766799997782,20.16528398573,21.1538879716818,21.9911485751285),
 .UNSPECIFIED.);
#360=B_SPLINE_CURVE_WITH_KNOTS('',3,(#17103,#17104,#17105,#17106,#17107,
#17108,#17109,#17110,#17111,#17112,#17113,#17114,#17115,#17116,#17117,#17118,
#17119,#17120,#17121,#17122,#17123,#17124,#17125,#17126,#17127,#17128,#17129,
#17130,#17131,#17132,#17133,#17134,#17135,#17136,#17137,#17138,#17139,#17140,
#17141,#17142,#17143,#17144,#17145,#17146,#17147,#17148,#17149,#17150,#17151,
#17152,#17153,#17154,#17155,#17156,#17157,#17158,#17159,#17160,#17161,#17162,
#17163,#17164,#17165,#17166,#17167,#17168,#17169,#17170,#17171,#17172,#17173,
#17174,#17175,#17176,#17177,#17178,#17179,#17180,#17181,#17182,#17183,#17184,
#17185,#17186,#17187),.UNSPECIFIED.,.F.,.F.,(4,3,3,3,3,3,3,3,3,3,3,3,3,
3,3,3,3,3,3,3,3,3,3,3,3,3,3,3,4),(-0.27663179171271,-0.2651301030347,-0.250460786414225,
-0.245045718144737,-0.241800530081285,-0.226536328657412,-0.215620637943102,
-0.212140369574972,-0.209334257433326,-0.193597942693264,-0.177548592082217,
-0.167964144797397,-0.163147554742663,-0.159540919290815,-0.14301553793474,
-0.139210802942938,-0.123238048148458,-0.115535670139179,-0.110632353224551,
-0.107705074830832,-0.0911577161793469,-0.074249565407069,-0.064760271735975,
-0.0583780708391448,-0.053731028480074,-0.0362740667018561,-0.018137033350928,
-0.00108826469303175,0.),.UNSPECIFIED.);
#361=B_SPLINE_CURVE_WITH_KNOTS('',3,(#17192,#17193,#17194,#17195,#17196,
#17197,#17198,#17199,#17200,#17201,#17202,#17203,#17204,#17205,#17206,#17207,
#17208,#17209,#17210,#17211,#17212,#17213,#17214,#17215,#17216,#17217,#17218,
#17219,#17220,#17221,#17222,#17223,#17224,#17225,#17226,#17227,#17228,#17229,
#17230,#17231,#17232,#17233,#17234,#17235,#17236,#17237,#17238,#17239,#17240,
#17241,#17242,#17243,#17244,#17245,#17246,#17247,#17248,#17249,#17250,#17251,
#17252,#17253,#17254,#17255,#17256,#17257,#17258,#17259,#17260,#17261,#17262,
#17263,#17264,#17265,#17266,#17267,#17268,#17269,#17270,#17271,#17272,#17273),
 .UNSPECIFIED.,.F.,.F.,(4,3,3,3,3,3,3,3,3,3,3,3,3,3,3,3,3,3,3,3,3,3,3,3,
3,3,3,4),(-0.275362278356885,-0.261358215039034,-0.24420947844022,-0.239226268528359,
-0.234169052699615,-0.216973772971366,-0.205373091631011,-0.200128212738553,
-0.196878691185682,-0.180126653267857,-0.163783011764808,-0.153879339385736,
-0.149003330340905,-0.145912671051637,-0.130035116133936,-0.124168322248522,
-0.108234162937227,-0.100893521573436,-0.0956516943326387,-0.0926034073274861,
-0.0768394523952997,-0.0611489821427944,-0.0532954156811162,-0.0475078582072449,
-0.0447093270180608,-0.0295993550201047,-0.0147996775100523,0.),
 .UNSPECIFIED.);
#362=B_SPLINE_CURVE_WITH_KNOTS('',3,(#17602,#17603,#17604,#17605,#17606,
#17607,#17608,#17609,#17610,#17611,#17612,#17613,#17614,#17615,#17616,#17617,
#17618,#17619,#17620),.UNSPECIFIED.,.F.,.F.,(4,3,3,3,3,3,4),(70.2377801854364,
71.1794869885301,72.1680909744818,73.1566949604337,74.1452989463855,75.1339029323373,
76.026542216873),.UNSPECIFIED.);
#363=B_SPLINE_CURVE_WITH_KNOTS('',3,(#17622,#17623,#17624,#17625,#17626,
#17627,#17628,#17629,#17630,#17631,#17632,#17633,#17634,#17635,#17636,#17637,
#17638,#17639,#17640,#17641,#17642,#17643,#17644,#17645,#17646,#17647,#17648,
#17649,#17650,#17651,#17652,#17653,#17654,#17655,#17656,#17657,#17658,#17659,
#17660,#17661,#17662,#17663,#17664,#17665,#17666,#17667,#17668,#17669,#17670,
#17671,#17672,#17673,#17674,#17675,#17676,#17677,#17678,#17679,#17680,#17681,
#17682,#17683,#17684,#17685,#17686,#17687,#17688,#17689,#17690,#17691,#17692,
#17693,#17694,#17695,#17696,#17697,#17698,#17699,#17700,#17701,#17702,#17703,
#17704,#17705,#17706),.UNSPECIFIED.,.F.,.F.,(4,3,3,3,3,3,3,3,3,3,3,3,3,
3,3,3,3,3,3,3,3,3,3,3,3,3,3,3,4),(-0.276631791712721,-0.265130103034713,
-0.250460792531934,-0.24504572637101,-0.241800547465848,-0.226536350695918,
-0.215620657226796,-0.212140587651992,-0.209334513885687,-0.193598209427458,
-0.177548857689101,-0.167964344002561,-0.163147689853096,-0.159540965946658,
-0.143015584324094,-0.139210802942942,-0.123238050693282,-0.115535672524952,
-0.110632355020678,-0.107705075837133,-0.0911577201523597,-0.0742495721522352,
-0.064760273687438,-0.0583780759534126,-0.0537310263259031,-0.0362740663814007,
-0.0181370331907004,-0.00108825577301921,0.),.UNSPECIFIED.);
#364=B_SPLINE_CURVE_WITH_KNOTS('',3,(#17707,#17708,#17709,#17710,#17711,
#17712,#17713,#17714,#17715),.UNSPECIFIED.,.F.,.F.,(4,1,1,1,1,1,4),(10.375208827628,
11.2678481121638,12.2564520981156,13.2450560840674,14.2336600700192,15.222264055971,
15.7079632679489),.UNSPECIFIED.);
#365=B_SPLINE_CURVE_WITH_KNOTS('',3,(#17721,#17722,#17723,#17724,#17725,
#17726,#17727,#17728,#17729,#17730,#17731,#17732,#17733,#17734,#17735,#17736,
#17737,#17738,#17739,#17740,#17741,#17742,#17743,#17744,#17745,#17746,#17747,
#17748,#17749,#17750,#17751,#17752,#17753,#17754,#17755,#17756,#17757,#17758,
#17759,#17760,#17761,#17762,#17763,#17764,#17765,#17766,#17767,#17768,#17769,
#17770,#17771,#17772,#17773,#17774,#17775,#17776,#17777,#17778,#17779,#17780,
#17781,#17782,#17783,#17784,#17785,#17786,#17787,#17788,#17789,#17790,#17791,
#17792,#17793,#17794,#17795,#17796,#17797,#17798,#17799,#17800,#17801,#17802),
 .UNSPECIFIED.,.F.,.F.,(4,3,3,3,3,3,3,3,3,3,3,3,3,3,3,3,3,3,3,3,3,3,3,3,
3,3,3,4),(-0.275362278356884,-0.26135821503903,-0.244209478440216,-0.239226264711111,
-0.234169052469442,-0.216973772681103,-0.20537309137703,-0.200128210040024,
-0.196878689389314,-0.180126650893078,-0.163783003806357,-0.153879333416897,
-0.149003310760071,-0.145912654690853,-0.130035094652386,-0.124168322248516,
-0.108234162817484,-0.100893518944725,-0.0956516935782954,-0.0926034075571851,
-0.0768394511997701,-0.061148985158665,-0.0532954165631934,-0.0475078611084516,
-0.0447093297178545,-0.0295993633295068,-0.0147996816647534,0.),
 .UNSPECIFIED.);
#366=B_SPLINE_CURVE_WITH_KNOTS('',3,(#17805,#17806,#17807,#17808,#17809,
#17810,#17811,#17812),.UNSPECIFIED.,.F.,.F.,(4,1,1,1,1,4),(11.6159397475004,
12.6045437334522,13.593147719404,14.5817517053558,15.5703556913076,15.7079632679489),
 .UNSPECIFIED.);
#367=B_SPLINE_CURVE_WITH_KNOTS('',3,(#18141,#18142,#18143,#18144,#18145,
#18146,#18147,#18148,#18149,#18150,#18151,#18152,#18153,#18154,#18155,#18156),
 .UNSPECIFIED.,.F.,.F.,(4,3,3,3,3,4),(-78.0997148901927,-77.1111109042409,
-76.1225069182891,-75.1339029323373,-74.1452989463855,-73.207061899424),
 .UNSPECIFIED.);
#432=CONICAL_SURFACE('',#9919,0.5,1.02242932542481);
#433=CONICAL_SURFACE('',#9930,1.35,0.785398163397448);
#434=CONICAL_SURFACE('',#9933,2.325,0.785398163397448);
#448=SHAPE_REPRESENTATION_RELATIONSHIP('SRR','None',#18350,#461);
#461=ADVANCED_BREP_SHAPE_REPRESENTATION('',(#492),#18279);
#479=STYLED_ITEM('',(#18481),#492);
#492=MANIFOLD_SOLID_BREP('Body1',#9096);
#552=CYLINDRICAL_SURFACE('',#9885,1.4635);
#553=CYLINDRICAL_SURFACE('',#9887,1.4635);
#554=CYLINDRICAL_SURFACE('',#9888,1.4635);
#555=CYLINDRICAL_SURFACE('',#9889,1.4635);
#556=CYLINDRICAL_SURFACE('',#9890,1.4635);
#557=CYLINDRICAL_SURFACE('',#9891,1.4635);
#558=CYLINDRICAL_SURFACE('',#9892,1.4635);
#559=CYLINDRICAL_SURFACE('',#9893,1.4635);
#560=CYLINDRICAL_SURFACE('',#9894,1.4635);
#561=CYLINDRICAL_SURFACE('',#9895,1.4635);
#562=CYLINDRICAL_SURFACE('',#9896,1.4635);
#563=CYLINDRICAL_SURFACE('',#9897,1.4635);
#564=CYLINDRICAL_SURFACE('',#9898,1.17775);
#565=CYLINDRICAL_SURFACE('',#9900,1.17775);
#566=CYLINDRICAL_SURFACE('',#9901,1.17775);
#567=CYLINDRICAL_SURFACE('',#9902,1.17775);
#568=CYLINDRICAL_SURFACE('',#9903,1.17775);
#569=CYLINDRICAL_SURFACE('',#9904,1.17775);
#570=CYLINDRICAL_SURFACE('',#9905,1.17775);
#571=CYLINDRICAL_SURFACE('',#9906,1.17775);
#572=CYLINDRICAL_SURFACE('',#9907,1.17775);
#573=CYLINDRICAL_SURFACE('',#9908,1.17775);
#574=CYLINDRICAL_SURFACE('',#9909,1.17775);
#575=CYLINDRICAL_SURFACE('',#9910,1.17775);
#576=CYLINDRICAL_SURFACE('',#9918,1.17775);
#577=CYLINDRICAL_SURFACE('',#9931,1.4635);
#627=FACE_BOUND('',#1924,.T.);
#628=FACE_BOUND('',#1930,.T.);
#807=CIRCLE('',#9886,1.4635);
#808=CIRCLE('',#9899,1.17775);
#809=CIRCLE('',#9912,1.4635);
#810=CIRCLE('',#9913,1.4635);
#811=CIRCLE('',#9915,1.4635);
#812=CIRCLE('',#9916,1.4635);
#813=CIRCLE('',#9917,1.17775);
#814=CIRCLE('',#9920,0.983629653494575);
#815=CIRCLE('',#9929,1.2);
#816=CIRCLE('',#9932,1.4635);
#817=CIRCLE('',#9934,3.15);
#1317=FACE_OUTER_BOUND('',#1887,.T.);
#1318=FACE_OUTER_BOUND('',#1888,.T.);
#1319=FACE_OUTER_BOUND('',#1889,.T.);
#1320=FACE_OUTER_BOUND('',#1890,.T.);
#1321=FACE_OUTER_BOUND('',#1891,.T.);
#1322=FACE_OUTER_BOUND('',#1892,.T.);
#1323=FACE_OUTER_BOUND('',#1893,.T.);
#1324=FACE_OUTER_BOUND('',#1894,.T.);
#1325=FACE_OUTER_BOUND('',#1895,.T.);
#1326=FACE_OUTER_BOUND('',#1896,.T.);
#1327=FACE_OUTER_BOUND('',#1897,.T.);
#1328=FACE_OUTER_BOUND('',#1898,.T.);
#1329=FACE_OUTER_BOUND('',#1899,.T.);
#1330=FACE_OUTER_BOUND('',#1900,.T.);
#1331=FACE_OUTER_BOUND('',#1901,.T.);
#1332=FACE_OUTER_BOUND('',#1902,.T.);
#1333=FACE_OUTER_BOUND('',#1903,.T.);
#1334=FACE_OUTER_BOUND('',#1904,.T.);
#1335=FACE_OUTER_BOUND('',#1905,.T.);
#1336=FACE_OUTER_BOUND('',#1906,.T.);
#1337=FACE_OUTER_BOUND('',#1907,.T.);
#1338=FACE_OUTER_BOUND('',#1908,.T.);
#1339=FACE_OUTER_BOUND('',#1909,.T.);
#1340=FACE_OUTER_BOUND('',#1910,.T.);
#1341=FACE_OUTER_BOUND('',#1911,.T.);
#1342=FACE_OUTER_BOUND('',#1912,.T.);
#1343=FACE_OUTER_BOUND('',#1913,.T.);
#1344=FACE_OUTER_BOUND('',#1914,.T.);
#1345=FACE_OUTER_BOUND('',#1915,.T.);
#1346=FACE_OUTER_BOUND('',#1916,.T.);
#1347=FACE_OUTER_BOUND('',#1917,.T.);
#1348=FACE_OUTER_BOUND('',#1918,.T.);
#1349=FACE_OUTER_BOUND('',#1919,.T.);
#1350=FACE_OUTER_BOUND('',#1920,.T.);
#1351=FACE_OUTER_BOUND('',#1921,.T.);
#1352=FACE_OUTER_BOUND('',#1922,.T.);
#1353=FACE_OUTER_BOUND('',#1923,.T.);
#1354=FACE_OUTER_BOUND('',#1925,.T.);
#1355=FACE_OUTER_BOUND('',#1926,.T.);
#1356=FACE_OUTER_BOUND('',#1927,.T.);
#1357=FACE_OUTER_BOUND('',#1928,.T.);
#1358=FACE_OUTER_BOUND('',#1929,.T.);
#1887=EDGE_LOOP('',(#8002,#8003,#8004,#8005));
#1888=EDGE_LOOP('',(#8006,#8007,#8008,#8009));
#1889=EDGE_LOOP('',(#8010,#8011,#8012,#8013));
#1890=EDGE_LOOP('',(#8014,#8015,#8016,#8017));
#1891=EDGE_LOOP('',(#8018,#8019,#8020,#8021));
#1892=EDGE_LOOP('',(#8022,#8023,#8024,#8025));
#1893=EDGE_LOOP('',(#8026,#8027,#8028,#8029));
#1894=EDGE_LOOP('',(#8030,#8031,#8032,#8033));
#1895=EDGE_LOOP('',(#8034,#8035,#8036,#8037));
#1896=EDGE_LOOP('',(#8038,#8039,#8040,#8041));
#1897=EDGE_LOOP('',(#8042,#8043,#8044,#8045));
#1898=EDGE_LOOP('',(#8046,#8047,#8048,#8049));
#1899=EDGE_LOOP('',(#8050,#8051,#8052,#8053));
#1900=EDGE_LOOP('',(#8054,#8055,#8056,#8057));
#1901=EDGE_LOOP('',(#8058,#8059,#8060,#8061));
#1902=EDGE_LOOP('',(#8062,#8063,#8064,#8065));
#1903=EDGE_LOOP('',(#8066,#8067,#8068,#8069));
#1904=EDGE_LOOP('',(#8070,#8071,#8072,#8073));
#1905=EDGE_LOOP('',(#8074,#8075,#8076,#8077));
#1906=EDGE_LOOP('',(#8078,#8079,#8080,#8081));
#1907=EDGE_LOOP('',(#8082,#8083,#8084,#8085));
#1908=EDGE_LOOP('',(#8086,#8087,#8088,#8089));
#1909=EDGE_LOOP('',(#8090,#8091,#8092,#8093));
#1910=EDGE_LOOP('',(#8094,#8095,#8096,#8097));
#1911=EDGE_LOOP('',(#8098,#8099,#8100,#8101,#8102));
#1912=EDGE_LOOP('',(#8103,#8104,#8105,#8106,#8107,#8108,#8109,#8110,#8111,
#8112,#8113,#8114,#8115,#8116,#8117,#8118,#8119,#8120,#8121,#8122,#8123,
#8124,#8125,#8126,#8127,#8128,#8129,#8130));
#1913=EDGE_LOOP('',(#8131,#8132,#8133,#8134,#8135));
#1914=EDGE_LOOP('',(#8136,#8137,#8138,#8139));
#1915=EDGE_LOOP('',(#8140,#8141,#8142,#8143,#8144,#8145,#8146,#8147,#8148,
#8149,#8150,#8151,#8152,#8153,#8154,#8155,#8156,#8157,#8158,#8159,#8160,
#8161,#8162,#8163,#8164,#8165,#8166,#8167));
#1916=EDGE_LOOP('',(#8168,#8169,#8170));
#1917=EDGE_LOOP('',(#8171,#8172,#8173,#8174));
#1918=EDGE_LOOP('',(#8175,#8176,#8177,#8178));
#1919=EDGE_LOOP('',(#8179,#8180,#8181,#8182));
#1920=EDGE_LOOP('',(#8183,#8184,#8185,#8186));
#1921=EDGE_LOOP('',(#8187,#8188,#8189,#8190));
#1922=EDGE_LOOP('',(#8191,#8192,#8193,#8194));
#1923=EDGE_LOOP('',(#8195,#8196,#8197,#8198,#8199,#8200));
#1924=EDGE_LOOP('',(#8201));
#1925=EDGE_LOOP('',(#8202));
#1926=EDGE_LOOP('',(#8203,#8204,#8205,#8206,#8207,#8208));
#1927=EDGE_LOOP('',(#8209,#8210,#8211,#8212));
#1928=EDGE_LOOP('',(#8213,#8214,#8215,#8216,#8217,#8218));
#1929=EDGE_LOOP('',(#8219));
#1930=EDGE_LOOP('',(#8220,#8221,#8222,#8223,#8224,#8225));
#2733=LINE('',#16238,#3578);
#2734=LINE('',#16262,#3579);
#2735=LINE('',#16310,#3580);
#2736=LINE('',#16358,#3581);
#2737=LINE('',#16412,#3582);
#2738=LINE('',#16460,#3583);
#2739=LINE('',#16508,#3584);
#2740=LINE('',#16562,#3585);
#2741=LINE('',#16610,#3586);
#2742=LINE('',#16658,#3587);
#2743=LINE('',#16712,#3588);
#2744=LINE('',#16760,#3589);
#2745=LINE('',#16814,#3590);
#2746=LINE('',#16832,#3591);
#2747=LINE('',#16857,#3592);
#2748=LINE('',#16882,#3593);
#2749=LINE('',#16907,#3594);
#2750=LINE('',#16932,#3595);
#2751=LINE('',#16956,#3596);
#2752=LINE('',#16981,#3597);
#2753=LINE('',#17006,#3598);
#2754=LINE('',#17030,#3599);
#2755=LINE('',#17055,#3600);
#2756=LINE('',#17080,#3601);
#2757=LINE('',#18160,#3602);
#2758=LINE('',#18165,#3603);
#2759=LINE('',#18167,#3604);
#2760=LINE('',#18169,#3605);
#2761=LINE('',#18170,#3606);
#2762=LINE('',#18173,#3607);
#2763=LINE('',#18175,#3608);
#2764=LINE('',#18176,#3609);
#2765=LINE('',#18179,#3610);
#2766=LINE('',#18181,#3611);
#2767=LINE('',#18182,#3612);
#2768=LINE('',#18185,#3613);
#2769=LINE('',#18187,#3614);
#2770=LINE('',#18188,#3615);
#2771=LINE('',#18191,#3616);
#2772=LINE('',#18193,#3617);
#2773=LINE('',#18194,#3618);
#2774=LINE('',#18196,#3619);
#2775=LINE('',#18197,#3620);
#2776=LINE('',#18203,#3621);
#2777=LINE('',#18209,#3622);
#3578=VECTOR('',#12055,1.5);
#3579=VECTOR('',#12060,1.5);
#3580=VECTOR('',#12063,1.5);
#3581=VECTOR('',#12066,1.5);
#3582=VECTOR('',#12069,1.5);
#3583=VECTOR('',#12072,1.5);
#3584=VECTOR('',#12075,1.5);
#3585=VECTOR('',#12078,1.5);
#3586=VECTOR('',#12081,1.5);
#3587=VECTOR('',#12084,1.5);
#3588=VECTOR('',#12087,1.5);
#3589=VECTOR('',#12090,1.5);
#3590=VECTOR('',#12093,1.17775);
#3591=VECTOR('',#12098,1.17775);
#3592=VECTOR('',#12101,1.17775);
#3593=VECTOR('',#12104,1.17775);
#3594=VECTOR('',#12107,1.17775);
#3595=VECTOR('',#12110,1.17775);
#3596=VECTOR('',#12113,1.17775);
#3597=VECTOR('',#12116,1.17775);
#3598=VECTOR('',#12119,1.17775);
#3599=VECTOR('',#12122,1.17775);
#3600=VECTOR('',#12125,1.17775);
#3601=VECTOR('',#12128,1.17775);
#3602=VECTOR('',#12147,0.5);
#3603=VECTOR('',#12152,10.);
#3604=VECTOR('',#12153,10.);
#3605=VECTOR('',#12154,10.);
#3606=VECTOR('',#12155,10.);
#3607=VECTOR('',#12158,10.);
#3608=VECTOR('',#12159,10.);
#3609=VECTOR('',#12160,10.);
#3610=VECTOR('',#12163,10.);
#3611=VECTOR('',#12164,10.);
#3612=VECTOR('',#12165,10.);
#3613=VECTOR('',#12168,10.);
#3614=VECTOR('',#12169,10.);
#3615=VECTOR('',#12170,10.);
#3616=VECTOR('',#12173,10.);
#3617=VECTOR('',#12174,10.);
#3618=VECTOR('',#12175,10.);
#3619=VECTOR('',#12178,10.);
#3620=VECTOR('',#12179,10.);
#3621=VECTOR('',#12188,1.35);
#3622=VECTOR('',#12197,2.325);
#4340=VERTEX_POINT('',#16236);
#4341=VERTEX_POINT('',#16237);
#4342=VERTEX_POINT('',#16239);
#4343=VERTEX_POINT('',#16250);
#4344=VERTEX_POINT('',#16260);
#4345=VERTEX_POINT('',#16261);
#4346=VERTEX_POINT('',#16308);
#4347=VERTEX_POINT('',#16309);
#4348=VERTEX_POINT('',#16356);
#4349=VERTEX_POINT('',#16357);
#4350=VERTEX_POINT('',#16410);
#4351=VERTEX_POINT('',#16411);
#4352=VERTEX_POINT('',#16458);
#4353=VERTEX_POINT('',#16459);
#4354=VERTEX_POINT('',#16506);
#4355=VERTEX_POINT('',#16507);
#4356=VERTEX_POINT('',#16560);
#4357=VERTEX_POINT('',#16561);
#4358=VERTEX_POINT('',#16608);
#4359=VERTEX_POINT('',#16609);
#4360=VERTEX_POINT('',#16656);
#4361=VERTEX_POINT('',#16657);
#4362=VERTEX_POINT('',#16710);
#4363=VERTEX_POINT('',#16711);
#4364=VERTEX_POINT('',#16758);
#4365=VERTEX_POINT('',#16759);
#4366=VERTEX_POINT('',#16812);
#4367=VERTEX_POINT('',#16813);
#4368=VERTEX_POINT('',#16815);
#4369=VERTEX_POINT('',#16822);
#4370=VERTEX_POINT('',#16830);
#4371=VERTEX_POINT('',#16831);
#4372=VERTEX_POINT('',#16855);
#4373=VERTEX_POINT('',#16856);
#4374=VERTEX_POINT('',#16880);
#4375=VERTEX_POINT('',#16881);
#4376=VERTEX_POINT('',#16905);
#4377=VERTEX_POINT('',#16906);
#4378=VERTEX_POINT('',#16930);
#4379=VERTEX_POINT('',#16931);
#4380=VERTEX_POINT('',#16954);
#4381=VERTEX_POINT('',#16955);
#4382=VERTEX_POINT('',#16979);
#4383=VERTEX_POINT('',#16980);
#4384=VERTEX_POINT('',#17004);
#4385=VERTEX_POINT('',#17005);
#4386=VERTEX_POINT('',#17028);
#4387=VERTEX_POINT('',#17029);
#4388=VERTEX_POINT('',#17053);
#4389=VERTEX_POINT('',#17054);
#4390=VERTEX_POINT('',#17078);
#4391=VERTEX_POINT('',#17079);
#4392=VERTEX_POINT('',#17102);
#4393=VERTEX_POINT('',#17188);
#4394=VERTEX_POINT('',#17190);
#4395=VERTEX_POINT('',#17621);
#4396=VERTEX_POINT('',#17717);
#4397=VERTEX_POINT('',#17720);
#4398=VERTEX_POINT('',#18158);
#4399=VERTEX_POINT('',#18159);
#4400=VERTEX_POINT('',#18163);
#4401=VERTEX_POINT('',#18164);
#4402=VERTEX_POINT('',#18166);
#4403=VERTEX_POINT('',#18168);
#4404=VERTEX_POINT('',#18172);
#4405=VERTEX_POINT('',#18174);
#4406=VERTEX_POINT('',#18178);
#4407=VERTEX_POINT('',#18180);
#4408=VERTEX_POINT('',#18184);
#4409=VERTEX_POINT('',#18186);
#4410=VERTEX_POINT('',#18190);
#4411=VERTEX_POINT('',#18192);
#4412=VERTEX_POINT('',#18200);
#4413=VERTEX_POINT('',#18207);
#5573=EDGE_CURVE('',#4340,#4341,#2733,.T.);
#5574=EDGE_CURVE('',#4340,#4342,#312,.T.);
#5575=EDGE_CURVE('',#4342,#4343,#807,.T.);
#5576=EDGE_CURVE('',#4343,#4341,#313,.T.);
#5577=EDGE_CURVE('',#4344,#4345,#2734,.T.);
#5578=EDGE_CURVE('',#4344,#4340,#314,.T.);
#5579=EDGE_CURVE('',#4341,#4345,#315,.T.);
#5580=EDGE_CURVE('',#4346,#4347,#2735,.T.);
#5581=EDGE_CURVE('',#4346,#4344,#316,.T.);
#5582=EDGE_CURVE('',#4345,#4347,#317,.T.);
#5583=EDGE_CURVE('',#4348,#4349,#2736,.T.);
#5584=EDGE_CURVE('',#4348,#4346,#318,.T.);
#5585=EDGE_CURVE('',#4347,#4349,#319,.T.);
#5586=EDGE_CURVE('',#4350,#4351,#2737,.T.);
#5587=EDGE_CURVE('',#4350,#4348,#320,.T.);
#5588=EDGE_CURVE('',#4349,#4351,#321,.T.);
#5589=EDGE_CURVE('',#4352,#4353,#2738,.T.);
#5590=EDGE_CURVE('',#4352,#4350,#322,.T.);
#5591=EDGE_CURVE('',#4351,#4353,#323,.T.);
#5592=EDGE_CURVE('',#4354,#4355,#2739,.T.);
#5593=EDGE_CURVE('',#4354,#4352,#324,.T.);
#5594=EDGE_CURVE('',#4353,#4355,#325,.T.);
#5595=EDGE_CURVE('',#4356,#4357,#2740,.T.);
#5596=EDGE_CURVE('',#4356,#4354,#326,.T.);
#5597=EDGE_CURVE('',#4355,#4357,#327,.T.);
#5598=EDGE_CURVE('',#4358,#4359,#2741,.T.);
#5599=EDGE_CURVE('',#4358,#4356,#328,.T.);
#5600=EDGE_CURVE('',#4357,#4359,#329,.T.);
#5601=EDGE_CURVE('',#4360,#4361,#2742,.T.);
#5602=EDGE_CURVE('',#4360,#4358,#330,.T.);
#5603=EDGE_CURVE('',#4359,#4361,#331,.T.);
#5604=EDGE_CURVE('',#4362,#4363,#2743,.T.);
#5605=EDGE_CURVE('',#4362,#4360,#332,.T.);
#5606=EDGE_CURVE('',#4361,#4363,#333,.T.);
#5607=EDGE_CURVE('',#4364,#4365,#2744,.T.);
#5608=EDGE_CURVE('',#4364,#4362,#334,.T.);
#5609=EDGE_CURVE('',#4363,#4365,#335,.T.);
#5610=EDGE_CURVE('',#4366,#4367,#2745,.T.);
#5611=EDGE_CURVE('',#4366,#4368,#336,.T.);
#5612=EDGE_CURVE('',#4369,#4368,#808,.T.);
#5613=EDGE_CURVE('',#4367,#4369,#337,.T.);
#5614=EDGE_CURVE('',#4370,#4371,#2746,.T.);
#5615=EDGE_CURVE('',#4370,#4366,#338,.T.);
#5616=EDGE_CURVE('',#4371,#4367,#339,.T.);
#5617=EDGE_CURVE('',#4372,#4373,#2747,.T.);
#5618=EDGE_CURVE('',#4372,#4370,#340,.T.);
#5619=EDGE_CURVE('',#4373,#4371,#341,.T.);
#5620=EDGE_CURVE('',#4374,#4375,#2748,.T.);
#5621=EDGE_CURVE('',#4374,#4372,#342,.T.);
#5622=EDGE_CURVE('',#4375,#4373,#343,.T.);
#5623=EDGE_CURVE('',#4376,#4377,#2749,.T.);
#5624=EDGE_CURVE('',#4376,#4374,#344,.T.);
#5625=EDGE_CURVE('',#4377,#4375,#345,.T.);
#5626=EDGE_CURVE('',#4378,#4379,#2750,.T.);
#5627=EDGE_CURVE('',#4378,#4376,#346,.T.);
#5628=EDGE_CURVE('',#4379,#4377,#347,.T.);
#5629=EDGE_CURVE('',#4380,#4381,#2751,.T.);
#5630=EDGE_CURVE('',#4380,#4378,#348,.T.);
#5631=EDGE_CURVE('',#4381,#4379,#349,.T.);
#5632=EDGE_CURVE('',#4382,#4383,#2752,.T.);
#5633=EDGE_CURVE('',#4382,#4380,#350,.T.);
#5634=EDGE_CURVE('',#4383,#4381,#351,.T.);
#5635=EDGE_CURVE('',#4384,#4385,#2753,.T.);
#5636=EDGE_CURVE('',#4384,#4382,#352,.T.);
#5637=EDGE_CURVE('',#4385,#4383,#353,.T.);
#5638=EDGE_CURVE('',#4386,#4387,#2754,.T.);
#5639=EDGE_CURVE('',#4386,#4384,#354,.T.);
#5640=EDGE_CURVE('',#4387,#4385,#355,.T.);
#5641=EDGE_CURVE('',#4388,#4389,#2755,.T.);
#5642=EDGE_CURVE('',#4388,#4386,#356,.T.);
#5643=EDGE_CURVE('',#4389,#4387,#357,.T.);
#5644=EDGE_CURVE('',#4390,#4391,#2756,.T.);
#5645=EDGE_CURVE('',#4390,#4388,#358,.T.);
#5646=EDGE_CURVE('',#4391,#4389,#359,.T.);
#5647=EDGE_CURVE('',#4368,#4392,#360,.T.);
#5648=EDGE_CURVE('',#4393,#4392,#809,.T.);
#5649=EDGE_CURVE('',#4394,#4393,#810,.T.);
#5650=EDGE_CURVE('',#4394,#4369,#361,.T.);
#5651=EDGE_CURVE('',#4365,#4394,#362,.T.);
#5652=EDGE_CURVE('',#4395,#4343,#363,.T.);
#5653=EDGE_CURVE('',#4395,#4391,#364,.T.);
#5654=EDGE_CURVE('',#4343,#4396,#811,.T.);
#5655=EDGE_CURVE('',#4396,#4342,#812,.T.);
#5656=EDGE_CURVE('',#4342,#4397,#365,.T.);
#5657=EDGE_CURVE('',#4397,#4395,#813,.T.);
#5658=EDGE_CURVE('',#4397,#4390,#366,.T.);
#5659=EDGE_CURVE('',#4392,#4364,#367,.T.);
#5660=EDGE_CURVE('',#4398,#4399,#2757,.T.);
#5661=EDGE_CURVE('',#4399,#4399,#814,.T.);
#5662=EDGE_CURVE('',#4400,#4401,#2758,.T.);
#5663=EDGE_CURVE('',#4400,#4402,#2759,.T.);
#5664=EDGE_CURVE('',#4402,#4403,#2760,.T.);
#5665=EDGE_CURVE('',#4401,#4403,#2761,.T.);
#5666=EDGE_CURVE('',#4404,#4400,#2762,.T.);
#5667=EDGE_CURVE('',#4404,#4405,#2763,.T.);
#5668=EDGE_CURVE('',#4405,#4402,#2764,.T.);
#5669=EDGE_CURVE('',#4406,#4404,#2765,.T.);
#5670=EDGE_CURVE('',#4406,#4407,#2766,.T.);
#5671=EDGE_CURVE('',#4407,#4405,#2767,.T.);
#5672=EDGE_CURVE('',#4408,#4406,#2768,.T.);
#5673=EDGE_CURVE('',#4408,#4409,#2769,.T.);
#5674=EDGE_CURVE('',#4409,#4407,#2770,.T.);
#5675=EDGE_CURVE('',#4410,#4408,#2771,.T.);
#5676=EDGE_CURVE('',#4410,#4411,#2772,.T.);
#5677=EDGE_CURVE('',#4411,#4409,#2773,.T.);
#5678=EDGE_CURVE('',#4401,#4410,#2774,.T.);
#5679=EDGE_CURVE('',#4403,#4411,#2775,.T.);
#5680=EDGE_CURVE('',#4412,#4412,#815,.T.);
#5681=EDGE_CURVE('',#4396,#4412,#2776,.T.);
#5682=EDGE_CURVE('',#4392,#4394,#816,.T.);
#5683=EDGE_CURVE('',#4413,#4413,#817,.T.);
#5684=EDGE_CURVE('',#4413,#4393,#2777,.T.);
#8002=ORIENTED_EDGE('',*,*,#5573,.F.);
#8003=ORIENTED_EDGE('',*,*,#5574,.T.);
#8004=ORIENTED_EDGE('',*,*,#5575,.T.);
#8005=ORIENTED_EDGE('',*,*,#5576,.T.);
#8006=ORIENTED_EDGE('',*,*,#5577,.F.);
#8007=ORIENTED_EDGE('',*,*,#5578,.T.);
#8008=ORIENTED_EDGE('',*,*,#5573,.T.);
#8009=ORIENTED_EDGE('',*,*,#5579,.T.);
#8010=ORIENTED_EDGE('',*,*,#5580,.F.);
#8011=ORIENTED_EDGE('',*,*,#5581,.T.);
#8012=ORIENTED_EDGE('',*,*,#5577,.T.);
#8013=ORIENTED_EDGE('',*,*,#5582,.T.);
#8014=ORIENTED_EDGE('',*,*,#5583,.F.);
#8015=ORIENTED_EDGE('',*,*,#5584,.T.);
#8016=ORIENTED_EDGE('',*,*,#5580,.T.);
#8017=ORIENTED_EDGE('',*,*,#5585,.T.);
#8018=ORIENTED_EDGE('',*,*,#5586,.F.);
#8019=ORIENTED_EDGE('',*,*,#5587,.T.);
#8020=ORIENTED_EDGE('',*,*,#5583,.T.);
#8021=ORIENTED_EDGE('',*,*,#5588,.T.);
#8022=ORIENTED_EDGE('',*,*,#5589,.F.);
#8023=ORIENTED_EDGE('',*,*,#5590,.T.);
#8024=ORIENTED_EDGE('',*,*,#5586,.T.);
#8025=ORIENTED_EDGE('',*,*,#5591,.T.);
#8026=ORIENTED_EDGE('',*,*,#5592,.F.);
#8027=ORIENTED_EDGE('',*,*,#5593,.T.);
#8028=ORIENTED_EDGE('',*,*,#5589,.T.);
#8029=ORIENTED_EDGE('',*,*,#5594,.T.);
#8030=ORIENTED_EDGE('',*,*,#5595,.F.);
#8031=ORIENTED_EDGE('',*,*,#5596,.T.);
#8032=ORIENTED_EDGE('',*,*,#5592,.T.);
#8033=ORIENTED_EDGE('',*,*,#5597,.T.);
#8034=ORIENTED_EDGE('',*,*,#5598,.F.);
#8035=ORIENTED_EDGE('',*,*,#5599,.T.);
#8036=ORIENTED_EDGE('',*,*,#5595,.T.);
#8037=ORIENTED_EDGE('',*,*,#5600,.T.);
#8038=ORIENTED_EDGE('',*,*,#5601,.F.);
#8039=ORIENTED_EDGE('',*,*,#5602,.T.);
#8040=ORIENTED_EDGE('',*,*,#5598,.T.);
#8041=ORIENTED_EDGE('',*,*,#5603,.T.);
#8042=ORIENTED_EDGE('',*,*,#5604,.F.);
#8043=ORIENTED_EDGE('',*,*,#5605,.T.);
#8044=ORIENTED_EDGE('',*,*,#5601,.T.);
#8045=ORIENTED_EDGE('',*,*,#5606,.T.);
#8046=ORIENTED_EDGE('',*,*,#5607,.F.);
#8047=ORIENTED_EDGE('',*,*,#5608,.T.);
#8048=ORIENTED_EDGE('',*,*,#5604,.T.);
#8049=ORIENTED_EDGE('',*,*,#5609,.T.);
#8050=ORIENTED_EDGE('',*,*,#5610,.F.);
#8051=ORIENTED_EDGE('',*,*,#5611,.T.);
#8052=ORIENTED_EDGE('',*,*,#5612,.F.);
#8053=ORIENTED_EDGE('',*,*,#5613,.F.);
#8054=ORIENTED_EDGE('',*,*,#5614,.F.);
#8055=ORIENTED_EDGE('',*,*,#5615,.T.);
#8056=ORIENTED_EDGE('',*,*,#5610,.T.);
#8057=ORIENTED_EDGE('',*,*,#5616,.F.);
#8058=ORIENTED_EDGE('',*,*,#5617,.F.);
#8059=ORIENTED_EDGE('',*,*,#5618,.T.);
#8060=ORIENTED_EDGE('',*,*,#5614,.T.);
#8061=ORIENTED_EDGE('',*,*,#5619,.F.);
#8062=ORIENTED_EDGE('',*,*,#5620,.F.);
#8063=ORIENTED_EDGE('',*,*,#5621,.T.);
#8064=ORIENTED_EDGE('',*,*,#5617,.T.);
#8065=ORIENTED_EDGE('',*,*,#5622,.F.);
#8066=ORIENTED_EDGE('',*,*,#5623,.F.);
#8067=ORIENTED_EDGE('',*,*,#5624,.T.);
#8068=ORIENTED_EDGE('',*,*,#5620,.T.);
#8069=ORIENTED_EDGE('',*,*,#5625,.F.);
#8070=ORIENTED_EDGE('',*,*,#5626,.F.);
#8071=ORIENTED_EDGE('',*,*,#5627,.T.);
#8072=ORIENTED_EDGE('',*,*,#5623,.T.);
#8073=ORIENTED_EDGE('',*,*,#5628,.F.);
#8074=ORIENTED_EDGE('',*,*,#5629,.F.);
#8075=ORIENTED_EDGE('',*,*,#5630,.T.);
#8076=ORIENTED_EDGE('',*,*,#5626,.T.);
#8077=ORIENTED_EDGE('',*,*,#5631,.F.);
#8078=ORIENTED_EDGE('',*,*,#5632,.F.);
#8079=ORIENTED_EDGE('',*,*,#5633,.T.);
#8080=ORIENTED_EDGE('',*,*,#5629,.T.);
#8081=ORIENTED_EDGE('',*,*,#5634,.F.);
#8082=ORIENTED_EDGE('',*,*,#5635,.F.);
#8083=ORIENTED_EDGE('',*,*,#5636,.T.);
#8084=ORIENTED_EDGE('',*,*,#5632,.T.);
#8085=ORIENTED_EDGE('',*,*,#5637,.F.);
#8086=ORIENTED_EDGE('',*,*,#5638,.F.);
#8087=ORIENTED_EDGE('',*,*,#5639,.T.);
#8088=ORIENTED_EDGE('',*,*,#5635,.T.);
#8089=ORIENTED_EDGE('',*,*,#5640,.F.);
#8090=ORIENTED_EDGE('',*,*,#5641,.F.);
#8091=ORIENTED_EDGE('',*,*,#5642,.T.);
#8092=ORIENTED_EDGE('',*,*,#5638,.T.);
#8093=ORIENTED_EDGE('',*,*,#5643,.F.);
#8094=ORIENTED_EDGE('',*,*,#5644,.F.);
#8095=ORIENTED_EDGE('',*,*,#5645,.T.);
#8096=ORIENTED_EDGE('',*,*,#5641,.T.);
#8097=ORIENTED_EDGE('',*,*,#5646,.F.);
#8098=ORIENTED_EDGE('',*,*,#5612,.T.);
#8099=ORIENTED_EDGE('',*,*,#5647,.T.);
#8100=ORIENTED_EDGE('',*,*,#5648,.F.);
#8101=ORIENTED_EDGE('',*,*,#5649,.F.);
#8102=ORIENTED_EDGE('',*,*,#5650,.T.);
#8103=ORIENTED_EDGE('',*,*,#5650,.F.);
#8104=ORIENTED_EDGE('',*,*,#5651,.F.);
#8105=ORIENTED_EDGE('',*,*,#5609,.F.);
#8106=ORIENTED_EDGE('',*,*,#5606,.F.);
#8107=ORIENTED_EDGE('',*,*,#5603,.F.);
#8108=ORIENTED_EDGE('',*,*,#5600,.F.);
#8109=ORIENTED_EDGE('',*,*,#5597,.F.);
#8110=ORIENTED_EDGE('',*,*,#5594,.F.);
#8111=ORIENTED_EDGE('',*,*,#5591,.F.);
#8112=ORIENTED_EDGE('',*,*,#5588,.F.);
#8113=ORIENTED_EDGE('',*,*,#5585,.F.);
#8114=ORIENTED_EDGE('',*,*,#5582,.F.);
#8115=ORIENTED_EDGE('',*,*,#5579,.F.);
#8116=ORIENTED_EDGE('',*,*,#5576,.F.);
#8117=ORIENTED_EDGE('',*,*,#5652,.F.);
#8118=ORIENTED_EDGE('',*,*,#5653,.T.);
#8119=ORIENTED_EDGE('',*,*,#5646,.T.);
#8120=ORIENTED_EDGE('',*,*,#5643,.T.);
#8121=ORIENTED_EDGE('',*,*,#5640,.T.);
#8122=ORIENTED_EDGE('',*,*,#5637,.T.);
#8123=ORIENTED_EDGE('',*,*,#5634,.T.);
#8124=ORIENTED_EDGE('',*,*,#5631,.T.);
#8125=ORIENTED_EDGE('',*,*,#5628,.T.);
#8126=ORIENTED_EDGE('',*,*,#5625,.T.);
#8127=ORIENTED_EDGE('',*,*,#5622,.T.);
#8128=ORIENTED_EDGE('',*,*,#5619,.T.);
#8129=ORIENTED_EDGE('',*,*,#5616,.T.);
#8130=ORIENTED_EDGE('',*,*,#5613,.T.);
#8131=ORIENTED_EDGE('',*,*,#5654,.T.);
#8132=ORIENTED_EDGE('',*,*,#5655,.T.);
#8133=ORIENTED_EDGE('',*,*,#5656,.T.);
#8134=ORIENTED_EDGE('',*,*,#5657,.T.);
#8135=ORIENTED_EDGE('',*,*,#5652,.T.);
#8136=ORIENTED_EDGE('',*,*,#5644,.T.);
#8137=ORIENTED_EDGE('',*,*,#5653,.F.);
#8138=ORIENTED_EDGE('',*,*,#5657,.F.);
#8139=ORIENTED_EDGE('',*,*,#5658,.T.);
#8140=ORIENTED_EDGE('',*,*,#5647,.F.);
#8141=ORIENTED_EDGE('',*,*,#5611,.F.);
#8142=ORIENTED_EDGE('',*,*,#5615,.F.);
#8143=ORIENTED_EDGE('',*,*,#5618,.F.);
#8144=ORIENTED_EDGE('',*,*,#5621,.F.);
#8145=ORIENTED_EDGE('',*,*,#5624,.F.);
#8146=ORIENTED_EDGE('',*,*,#5627,.F.);
#8147=ORIENTED_EDGE('',*,*,#5630,.F.);
#8148=ORIENTED_EDGE('',*,*,#5633,.F.);
#8149=ORIENTED_EDGE('',*,*,#5636,.F.);
#8150=ORIENTED_EDGE('',*,*,#5639,.F.);
#8151=ORIENTED_EDGE('',*,*,#5642,.F.);
#8152=ORIENTED_EDGE('',*,*,#5645,.F.);
#8153=ORIENTED_EDGE('',*,*,#5658,.F.);
#8154=ORIENTED_EDGE('',*,*,#5656,.F.);
#8155=ORIENTED_EDGE('',*,*,#5574,.F.);
#8156=ORIENTED_EDGE('',*,*,#5578,.F.);
#8157=ORIENTED_EDGE('',*,*,#5581,.F.);
#8158=ORIENTED_EDGE('',*,*,#5584,.F.);
#8159=ORIENTED_EDGE('',*,*,#5587,.F.);
#8160=ORIENTED_EDGE('',*,*,#5590,.F.);
#8161=ORIENTED_EDGE('',*,*,#5593,.F.);
#8162=ORIENTED_EDGE('',*,*,#5596,.F.);
#8163=ORIENTED_EDGE('',*,*,#5599,.F.);
#8164=ORIENTED_EDGE('',*,*,#5602,.F.);
#8165=ORIENTED_EDGE('',*,*,#5605,.F.);
#8166=ORIENTED_EDGE('',*,*,#5608,.F.);
#8167=ORIENTED_EDGE('',*,*,#5659,.F.);
#8168=ORIENTED_EDGE('',*,*,#5660,.T.);
#8169=ORIENTED_EDGE('',*,*,#5661,.F.);
#8170=ORIENTED_EDGE('',*,*,#5660,.F.);
#8171=ORIENTED_EDGE('',*,*,#5662,.F.);
#8172=ORIENTED_EDGE('',*,*,#5663,.T.);
#8173=ORIENTED_EDGE('',*,*,#5664,.T.);
#8174=ORIENTED_EDGE('',*,*,#5665,.F.);
#8175=ORIENTED_EDGE('',*,*,#5666,.F.);
#8176=ORIENTED_EDGE('',*,*,#5667,.T.);
#8177=ORIENTED_EDGE('',*,*,#5668,.T.);
#8178=ORIENTED_EDGE('',*,*,#5663,.F.);
#8179=ORIENTED_EDGE('',*,*,#5669,.F.);
#8180=ORIENTED_EDGE('',*,*,#5670,.T.);
#8181=ORIENTED_EDGE('',*,*,#5671,.T.);
#8182=ORIENTED_EDGE('',*,*,#5667,.F.);
#8183=ORIENTED_EDGE('',*,*,#5672,.F.);
#8184=ORIENTED_EDGE('',*,*,#5673,.T.);
#8185=ORIENTED_EDGE('',*,*,#5674,.T.);
#8186=ORIENTED_EDGE('',*,*,#5670,.F.);
#8187=ORIENTED_EDGE('',*,*,#5675,.F.);
#8188=ORIENTED_EDGE('',*,*,#5676,.T.);
#8189=ORIENTED_EDGE('',*,*,#5677,.T.);
#8190=ORIENTED_EDGE('',*,*,#5673,.F.);
#8191=ORIENTED_EDGE('',*,*,#5678,.F.);
#8192=ORIENTED_EDGE('',*,*,#5665,.T.);
#8193=ORIENTED_EDGE('',*,*,#5679,.T.);
#8194=ORIENTED_EDGE('',*,*,#5676,.F.);
#8195=ORIENTED_EDGE('',*,*,#5679,.F.);
#8196=ORIENTED_EDGE('',*,*,#5664,.F.);
#8197=ORIENTED_EDGE('',*,*,#5668,.F.);
#8198=ORIENTED_EDGE('',*,*,#5671,.F.);
#8199=ORIENTED_EDGE('',*,*,#5674,.F.);
#8200=ORIENTED_EDGE('',*,*,#5677,.F.);
#8201=ORIENTED_EDGE('',*,*,#5661,.T.);
#8202=ORIENTED_EDGE('',*,*,#5680,.F.);
#8203=ORIENTED_EDGE('',*,*,#5654,.F.);
#8204=ORIENTED_EDGE('',*,*,#5575,.F.);
#8205=ORIENTED_EDGE('',*,*,#5655,.F.);
#8206=ORIENTED_EDGE('',*,*,#5681,.T.);
#8207=ORIENTED_EDGE('',*,*,#5680,.T.);
#8208=ORIENTED_EDGE('',*,*,#5681,.F.);
#8209=ORIENTED_EDGE('',*,*,#5607,.T.);
#8210=ORIENTED_EDGE('',*,*,#5651,.T.);
#8211=ORIENTED_EDGE('',*,*,#5682,.F.);
#8212=ORIENTED_EDGE('',*,*,#5659,.T.);
#8213=ORIENTED_EDGE('',*,*,#5683,.F.);
#8214=ORIENTED_EDGE('',*,*,#5684,.T.);
#8215=ORIENTED_EDGE('',*,*,#5648,.T.);
#8216=ORIENTED_EDGE('',*,*,#5682,.T.);
#8217=ORIENTED_EDGE('',*,*,#5649,.T.);
#8218=ORIENTED_EDGE('',*,*,#5684,.F.);
#8219=ORIENTED_EDGE('',*,*,#5683,.T.);
#8220=ORIENTED_EDGE('',*,*,#5662,.T.);
#8221=ORIENTED_EDGE('',*,*,#5678,.T.);
#8222=ORIENTED_EDGE('',*,*,#5675,.T.);
#8223=ORIENTED_EDGE('',*,*,#5672,.T.);
#8224=ORIENTED_EDGE('',*,*,#5669,.T.);
#8225=ORIENTED_EDGE('',*,*,#5666,.T.);
#8550=PLANE('',#9911);
#8551=PLANE('',#9914);
#8552=PLANE('',#9921);
#8553=PLANE('',#9922);
#8554=PLANE('',#9923);
#8555=PLANE('',#9924);
#8556=PLANE('',#9925);
#8557=PLANE('',#9926);
#8558=PLANE('',#9927);
#8559=PLANE('',#9928);
#8560=PLANE('',#9935);
#9038=ADVANCED_FACE('',(#1317),#552,.T.);
#9039=ADVANCED_FACE('',(#1318),#553,.T.);
#9040=ADVANCED_FACE('',(#1319),#554,.T.);
#9041=ADVANCED_FACE('',(#1320),#555,.T.);
#9042=ADVANCED_FACE('',(#1321),#556,.T.);
#9043=ADVANCED_FACE('',(#1322),#557,.T.);
#9044=ADVANCED_FACE('',(#1323),#558,.T.);
#9045=ADVANCED_FACE('',(#1324),#559,.T.);
#9046=ADVANCED_FACE('',(#1325),#560,.T.);
#9047=ADVANCED_FACE('',(#1326),#561,.T.);
#9048=ADVANCED_FACE('',(#1327),#562,.T.);
#9049=ADVANCED_FACE('',(#1328),#563,.T.);
#9050=ADVANCED_FACE('',(#1329),#564,.T.);
#9051=ADVANCED_FACE('',(#1330),#565,.T.);
#9052=ADVANCED_FACE('',(#1331),#566,.T.);
#9053=ADVANCED_FACE('',(#1332),#567,.T.);
#9054=ADVANCED_FACE('',(#1333),#568,.T.);
#9055=ADVANCED_FACE('',(#1334),#569,.T.);
#9056=ADVANCED_FACE('',(#1335),#570,.T.);
#9057=ADVANCED_FACE('',(#1336),#571,.T.);
#9058=ADVANCED_FACE('',(#1337),#572,.T.);
#9059=ADVANCED_FACE('',(#1338),#573,.T.);
#9060=ADVANCED_FACE('',(#1339),#574,.T.);
#9061=ADVANCED_FACE('',(#1340),#575,.T.);
#9062=ADVANCED_FACE('',(#1341),#8550,.F.);
#9063=ADVANCED_FACE('',(#1342),#186,.F.);
#9064=ADVANCED_FACE('',(#1343),#8551,.T.);
#9065=ADVANCED_FACE('',(#1344),#576,.T.);
#9066=ADVANCED_FACE('',(#1345),#187,.F.);
#9067=ADVANCED_FACE('',(#1346),#432,.F.);
#9068=ADVANCED_FACE('',(#1347),#8552,.F.);
#9069=ADVANCED_FACE('',(#1348),#8553,.F.);
#9070=ADVANCED_FACE('',(#1349),#8554,.F.);
#9071=ADVANCED_FACE('',(#1350),#8555,.F.);
#9072=ADVANCED_FACE('',(#1351),#8556,.F.);
#9073=ADVANCED_FACE('',(#1352),#8557,.F.);
#9074=ADVANCED_FACE('',(#1353,#627),#8558,.F.);
#9075=ADVANCED_FACE('',(#1354),#8559,.T.);
#9076=ADVANCED_FACE('',(#1355),#433,.T.);
#9077=ADVANCED_FACE('',(#1356),#577,.T.);
#9078=ADVANCED_FACE('',(#1357),#434,.T.);
#9079=ADVANCED_FACE('',(#1358,#628),#8560,.T.);
#9096=CLOSED_SHELL('',(#9038,#9039,#9040,#9041,#9042,#9043,#9044,#9045,
#9046,#9047,#9048,#9049,#9050,#9051,#9052,#9053,#9054,#9055,#9056,#9057,
#9058,#9059,#9060,#9061,#9062,#9063,#9064,#9065,#9066,#9067,#9068,#9069,
#9070,#9071,#9072,#9073,#9074,#9075,#9076,#9077,#9078,#9079));
#9884=AXIS2_PLACEMENT_3D('',#16234,#12051,#12052);
#9885=AXIS2_PLACEMENT_3D('',#16235,#12053,#12054);
#9886=AXIS2_PLACEMENT_3D('',#16251,#12056,#12057);
#9887=AXIS2_PLACEMENT_3D('',#16259,#12058,#12059);
#9888=AXIS2_PLACEMENT_3D('',#16307,#12061,#12062);
#9889=AXIS2_PLACEMENT_3D('',#16355,#12064,#12065);
#9890=AXIS2_PLACEMENT_3D('',#16409,#12067,#12068);
#9891=AXIS2_PLACEMENT_3D('',#16457,#12070,#12071);
#9892=AXIS2_PLACEMENT_3D('',#16505,#12073,#12074);
#9893=AXIS2_PLACEMENT_3D('',#16559,#12076,#12077);
#9894=AXIS2_PLACEMENT_3D('',#16607,#12079,#12080);
#9895=AXIS2_PLACEMENT_3D('',#16655,#12082,#12083);
#9896=AXIS2_PLACEMENT_3D('',#16709,#12085,#12086);
#9897=AXIS2_PLACEMENT_3D('',#16757,#12088,#12089);
#9898=AXIS2_PLACEMENT_3D('',#16811,#12091,#12092);
#9899=AXIS2_PLACEMENT_3D('',#16823,#12094,#12095);
#9900=AXIS2_PLACEMENT_3D('',#16829,#12096,#12097);
#9901=AXIS2_PLACEMENT_3D('',#16854,#12099,#12100);
#9902=AXIS2_PLACEMENT_3D('',#16879,#12102,#12103);
#9903=AXIS2_PLACEMENT_3D('',#16904,#12105,#12106);
#9904=AXIS2_PLACEMENT_3D('',#16929,#12108,#12109);
#9905=AXIS2_PLACEMENT_3D('',#16953,#12111,#12112);
#9906=AXIS2_PLACEMENT_3D('',#16978,#12114,#12115);
#9907=AXIS2_PLACEMENT_3D('',#17003,#12117,#12118);
#9908=AXIS2_PLACEMENT_3D('',#17027,#12120,#12121);
#9909=AXIS2_PLACEMENT_3D('',#17052,#12123,#12124);
#9910=AXIS2_PLACEMENT_3D('',#17077,#12126,#12127);
#9911=AXIS2_PLACEMENT_3D('',#17101,#12129,#12130);
#9912=AXIS2_PLACEMENT_3D('',#17189,#12131,#12132);
#9913=AXIS2_PLACEMENT_3D('',#17191,#12133,#12134);
#9914=AXIS2_PLACEMENT_3D('',#17716,#12135,#12136);
#9915=AXIS2_PLACEMENT_3D('',#17718,#12137,#12138);
#9916=AXIS2_PLACEMENT_3D('',#17719,#12139,#12140);
#9917=AXIS2_PLACEMENT_3D('',#17803,#12141,#12142);
#9918=AXIS2_PLACEMENT_3D('',#17804,#12143,#12144);
#9919=AXIS2_PLACEMENT_3D('',#18157,#12145,#12146);
#9920=AXIS2_PLACEMENT_3D('',#18161,#12148,#12149);
#9921=AXIS2_PLACEMENT_3D('',#18162,#12150,#12151);
#9922=AXIS2_PLACEMENT_3D('',#18171,#12156,#12157);
#9923=AXIS2_PLACEMENT_3D('',#18177,#12161,#12162);
#9924=AXIS2_PLACEMENT_3D('',#18183,#12166,#12167);
#9925=AXIS2_PLACEMENT_3D('',#18189,#12171,#12172);
#9926=AXIS2_PLACEMENT_3D('',#18195,#12176,#12177);
#9927=AXIS2_PLACEMENT_3D('',#18198,#12180,#12181);
#9928=AXIS2_PLACEMENT_3D('',#18199,#12182,#12183);
#9929=AXIS2_PLACEMENT_3D('',#18201,#12184,#12185);
#9930=AXIS2_PLACEMENT_3D('',#18202,#12186,#12187);
#9931=AXIS2_PLACEMENT_3D('',#18204,#12189,#12190);
#9932=AXIS2_PLACEMENT_3D('',#18205,#12191,#12192);
#9933=AXIS2_PLACEMENT_3D('',#18206,#12193,#12194);
#9934=AXIS2_PLACEMENT_3D('',#18208,#12195,#12196);
#9935=AXIS2_PLACEMENT_3D('',#18210,#12198,#12199);
#12051=DIRECTION('axis',(0.,0.,1.));
#12052=DIRECTION('refdir',(1.,0.,0.));
#12053=DIRECTION('center_axis',(1.,0.,0.));
#12054=DIRECTION('ref_axis',(0.,1.,0.));
#12055=DIRECTION('',(-1.,0.,0.));
#12056=DIRECTION('center_axis',(1.,0.,0.));
#12057=DIRECTION('ref_axis',(0.,1.,0.));
#12058=DIRECTION('center_axis',(1.,0.,0.));
#12059=DIRECTION('ref_axis',(0.,1.,0.));
#12060=DIRECTION('',(-1.,0.,0.));
#12061=DIRECTION('center_axis',(1.,0.,0.));
#12062=DIRECTION('ref_axis',(0.,1.,0.));
#12063=DIRECTION('',(-1.,0.,0.));
#12064=DIRECTION('center_axis',(1.,0.,0.));
#12065=DIRECTION('ref_axis',(0.,1.,0.));
#12066=DIRECTION('',(-1.,0.,0.));
#12067=DIRECTION('center_axis',(1.,0.,0.));
#12068=DIRECTION('ref_axis',(0.,1.,0.));
#12069=DIRECTION('',(-1.,0.,0.));
#12070=DIRECTION('center_axis',(1.,0.,0.));
#12071=DIRECTION('ref_axis',(0.,1.,0.));
#12072=DIRECTION('',(-1.,0.,0.));
#12073=DIRECTION('center_axis',(1.,0.,0.));
#12074=DIRECTION('ref_axis',(0.,1.,0.));
#12075=DIRECTION('',(-1.,0.,0.));
#12076=DIRECTION('center_axis',(1.,0.,0.));
#12077=DIRECTION('ref_axis',(0.,1.,0.));
#12078=DIRECTION('',(-1.,0.,0.));
#12079=DIRECTION('center_axis',(1.,0.,0.));
#12080=DIRECTION('ref_axis',(0.,1.,0.));
#12081=DIRECTION('',(-1.,0.,0.));
#12082=DIRECTION('center_axis',(1.,0.,0.));
#12083=DIRECTION('ref_axis',(0.,1.,0.));
#12084=DIRECTION('',(-1.,0.,0.));
#12085=DIRECTION('center_axis',(1.,0.,0.));
#12086=DIRECTION('ref_axis',(0.,1.,0.));
#12087=DIRECTION('',(-1.,0.,0.));
#12088=DIRECTION('center_axis',(1.,0.,0.));
#12089=DIRECTION('ref_axis',(0.,1.,0.));
#12090=DIRECTION('',(-1.,0.,0.));
#12091=DIRECTION('center_axis',(1.,0.,0.));
#12092=DIRECTION('ref_axis',(0.,-0.160289682943514,-0.987070016534728));
#12093=DIRECTION('',(1.,0.,0.));
#12094=DIRECTION('center_axis',(1.,0.,0.));
#12095=DIRECTION('ref_axis',(0.,1.,7.97687035098722E-14));
#12096=DIRECTION('center_axis',(1.,0.,0.));
#12097=DIRECTION('ref_axis',(0.,1.,7.97687035098722E-14));
#12098=DIRECTION('',(1.,0.,0.));
#12099=DIRECTION('center_axis',(1.,0.,0.));
#12100=DIRECTION('ref_axis',(0.,1.,7.97687035098722E-14));
#12101=DIRECTION('',(1.,0.,0.));
#12102=DIRECTION('center_axis',(1.,0.,0.));
#12103=DIRECTION('ref_axis',(0.,1.,7.97687035098722E-14));
#12104=DIRECTION('',(1.,0.,0.));
#12105=DIRECTION('center_axis',(1.,0.,0.));
#12106=DIRECTION('ref_axis',(0.,1.,7.97687035098722E-14));
#12107=DIRECTION('',(1.,0.,0.));
#12108=DIRECTION('center_axis',(1.,0.,0.));
#12109=DIRECTION('ref_axis',(0.,1.,7.97687035098722E-14));
#12110=DIRECTION('',(1.,0.,0.));
#12111=DIRECTION('center_axis',(1.,0.,0.));
#12112=DIRECTION('ref_axis',(0.,1.,7.97687035098722E-14));
#12113=DIRECTION('',(1.,0.,0.));
#12114=DIRECTION('center_axis',(1.,0.,0.));
#12115=DIRECTION('ref_axis',(0.,1.,7.97687035098722E-14));
#12116=DIRECTION('',(1.,0.,0.));
#12117=DIRECTION('center_axis',(1.,0.,0.));
#12118=DIRECTION('ref_axis',(0.,1.,7.97687035098722E-14));
#12119=DIRECTION('',(1.,0.,0.));
#12120=DIRECTION('center_axis',(1.,0.,0.));
#12121=DIRECTION('ref_axis',(0.,1.,7.97687035098722E-14));
#12122=DIRECTION('',(1.,0.,0.));
#12123=DIRECTION('center_axis',(1.,0.,0.));
#12124=DIRECTION('ref_axis',(0.,1.,7.97687035098722E-14));
#12125=DIRECTION('',(1.,0.,0.));
#12126=DIRECTION('center_axis',(1.,0.,0.));
#12127=DIRECTION('ref_axis',(0.,1.,7.97687035098722E-14));
#12128=DIRECTION('',(1.,0.,0.));
#12129=DIRECTION('center_axis',(1.,0.,0.));
#12130=DIRECTION('ref_axis',(0.,0.,-1.));
#12131=DIRECTION('center_axis',(1.,0.,0.));
#12132=DIRECTION('ref_axis',(0.,1.,0.));
#12133=DIRECTION('center_axis',(1.,0.,0.));
#12134=DIRECTION('ref_axis',(0.,1.,0.));
#12135=DIRECTION('center_axis',(1.,0.,0.));
#12136=DIRECTION('ref_axis',(0.,0.,-1.));
#12137=DIRECTION('center_axis',(1.,0.,0.));
#12138=DIRECTION('ref_axis',(0.,1.,0.));
#12139=DIRECTION('center_axis',(1.,0.,0.));
#12140=DIRECTION('ref_axis',(0.,1.,0.));
#12141=DIRECTION('center_axis',(-1.,0.,0.));
#12142=DIRECTION('ref_axis',(0.,1.,7.97687035098722E-14));
#12143=DIRECTION('center_axis',(1.,0.,0.));
#12144=DIRECTION('ref_axis',(0.,1.,7.97687035098722E-14));
#12145=DIRECTION('center_axis',(1.,0.,0.));
#12146=DIRECTION('ref_axis',(0.,1.,0.));
#12147=DIRECTION('',(0.521294361252099,-0.853376932502142,-1.04508532885494E-16));
#12148=DIRECTION('center_axis',(-1.,0.,0.));
#12149=DIRECTION('ref_axis',(0.,1.,0.));
#12150=DIRECTION('center_axis',(0.,0.5,0.866025403784439));
#12151=DIRECTION('ref_axis',(0.,0.866025403784439,-0.5));
#12152=DIRECTION('',(0.,0.866025403784439,-0.5));
#12153=DIRECTION('',(-1.,0.,0.));
#12154=DIRECTION('',(0.,0.866025403784439,-0.5));
#12155=DIRECTION('',(-1.,0.,0.));
#12156=DIRECTION('center_axis',(0.,-0.5,0.866025403784439));
#12157=DIRECTION('ref_axis',(0.,0.866025403784439,0.5));
#12158=DIRECTION('',(0.,0.866025403784439,0.5));
#12159=DIRECTION('',(-1.,0.,0.));
#12160=DIRECTION('',(0.,0.866025403784439,0.5));
#12161=DIRECTION('center_axis',(0.,-1.,-1.20185167898973E-16));
#12162=DIRECTION('ref_axis',(0.,-1.20185167898973E-16,1.));
#12163=DIRECTION('',(0.,-1.20185167898973E-16,1.));
#12164=DIRECTION('',(-1.,0.,0.));
#12165=DIRECTION('',(0.,-1.20185167898973E-16,1.));
#12166=DIRECTION('center_axis',(0.,-0.5,-0.866025403784439));
#12167=DIRECTION('ref_axis',(0.,-0.866025403784439,0.5));
#12168=DIRECTION('',(0.,-0.866025403784439,0.5));
#12169=DIRECTION('',(-1.,0.,0.));
#12170=DIRECTION('',(0.,-0.866025403784439,0.5));
#12171=DIRECTION('center_axis',(0.,0.5,-0.866025403784439));
#12172=DIRECTION('ref_axis',(0.,-0.866025403784439,-0.5));
#12173=DIRECTION('',(0.,-0.866025403784439,-0.5));
#12174=DIRECTION('',(-1.,0.,0.));
#12175=DIRECTION('',(0.,-0.866025403784439,-0.5));
#12176=DIRECTION('center_axis',(0.,1.,-3.60555503696918E-16));
#12177=DIRECTION('ref_axis',(0.,-3.60555503696918E-16,-1.));
#12178=DIRECTION('',(0.,-3.60555503696918E-16,-1.));
#12179=DIRECTION('',(0.,-3.60555503696918E-16,-1.));
#12180=DIRECTION('center_axis',(-1.,0.,0.));
#12181=DIRECTION('ref_axis',(0.,0.,1.));
#12182=DIRECTION('center_axis',(-1.,0.,0.));
#12183=DIRECTION('ref_axis',(0.,0.,1.));
#12184=DIRECTION('center_axis',(1.,0.,0.));
#12185=DIRECTION('ref_axis',(0.,0.,-1.));
#12186=DIRECTION('center_axis',(1.,0.,0.));
#12187=DIRECTION('ref_axis',(0.,1.,0.));
#12188=DIRECTION('',(-0.707106781186548,0.707106781186547,8.65956056235493E-17));
#12189=DIRECTION('center_axis',(1.,0.,0.));
#12190=DIRECTION('ref_axis',(0.,0.969617468264477,-0.244626174471142));
#12191=DIRECTION('center_axis',(1.,0.,0.));
#12192=DIRECTION('ref_axis',(0.,1.,0.));
#12193=DIRECTION('center_axis',(1.,0.,0.));
#12194=DIRECTION('ref_axis',(0.,1.,0.));
#12195=DIRECTION('center_axis',(1.,0.,0.));
#12196=DIRECTION('ref_axis',(0.,0.,-1.));
#12197=DIRECTION('',(-0.707106781186548,0.707106781186548,8.65956056235494E-17));
#12198=DIRECTION('center_axis',(1.,0.,0.));
#12199=DIRECTION('ref_axis',(0.,0.,-1.));
#16234=CARTESIAN_POINT('',(0.,0.,0.));
#16235=CARTESIAN_POINT('Origin',(-4.675,0.,0.));
#16236=CARTESIAN_POINT('',(-7.57584495415709,-1.46476825295553,0.00111815863164652));
#16237=CARTESIAN_POINT('',(-7.64715504584291,-1.46461339238561,0.00160511507277402));
#16238=CARTESIAN_POINT('',(-4.675,-1.4635,-1.79227059055215E-16));
#16239=CARTESIAN_POINT('',(-7.7365,0.63476680905654,1.31983838594169));
#16240=CARTESIAN_POINT('Ctrl Pts',(-7.57584495415709,-1.46476825295553,
0.00111815863164652));
#16241=CARTESIAN_POINT('Ctrl Pts',(-7.57949510849532,-1.46530187760278,
0.0680739723037402));
#16242=CARTESIAN_POINT('Ctrl Pts',(-7.58314526283355,-1.4611010846802,0.134958986929198));
#16243=CARTESIAN_POINT('Ctrl Pts',(-7.58679541717177,-1.45193482378899,
0.201151768713104));
#16244=CARTESIAN_POINT('Ctrl Pts',(-7.6130189523592,-1.38608233023814,0.676695699578037));
#16245=CARTESIAN_POINT('Ctrl Pts',(-7.63924248754663,-1.06394659683228,
1.11651134128917));
#16246=CARTESIAN_POINT('Ctrl Pts',(-7.66546602273406,-0.630444354550018,
1.32315907101614));
#16247=CARTESIAN_POINT('Ctrl Pts',(-7.68914401515605,-0.239022575056683,
1.50974731487885));
#16248=CARTESIAN_POINT('Ctrl Pts',(-7.71282200757803,0.243194194034392,
1.50623820939729));
#16249=CARTESIAN_POINT('Ctrl Pts',(-7.7365,0.635526523537879,1.32063649424652));
#16250=CARTESIAN_POINT('',(-7.7365,-0.634007094575234,1.31904027763684));
#16251=CARTESIAN_POINT('Origin',(-7.7365,0.,0.));
#16252=CARTESIAN_POINT('Ctrl Pts',(-7.7365,-0.634007094575232,1.31904027763684));
#16253=CARTESIAN_POINT('Ctrl Pts',(-7.71027646481257,-1.06867658660948,
1.11011296403058));
#16254=CARTESIAN_POINT('Ctrl Pts',(-7.68405292962514,-1.38849610006321,
0.67151411483421));
#16255=CARTESIAN_POINT('Ctrl Pts',(-7.65782939443771,-1.45248317015234,
0.196425540089081));
#16256=CARTESIAN_POINT('Ctrl Pts',(-7.65427127823944,-1.46116519677219,
0.13196358477567));
#16257=CARTESIAN_POINT('Ctrl Pts',(-7.65071316204118,-1.46513730485639,
0.0668298474456289));
#16258=CARTESIAN_POINT('Ctrl Pts',(-7.64715504584291,-1.46461339238561,
0.00160511507277402));
#16259=CARTESIAN_POINT('Origin',(-4.675,0.,0.));
#16260=CARTESIAN_POINT('',(-7.07584495415709,-1.46119452374026,4.09982538755738E-5));
#16261=CARTESIAN_POINT('',(-7.14715504584291,-1.46119347856455,7.51979904560513E-5));
#16262=CARTESIAN_POINT('',(-4.675,-1.4635,-1.79227059055215E-16));
#16263=CARTESIAN_POINT('Ctrl Pts',(-7.07584495415709,-1.46119452374026,
4.09982538755738E-5));
#16264=CARTESIAN_POINT('Ctrl Pts',(-7.0888205640374,-1.46125337597131,0.239559405180254));
#16265=CARTESIAN_POINT('Ctrl Pts',(-7.10179617391772,-1.40553952388032,
0.479051677557368));
#16266=CARTESIAN_POINT('Ctrl Pts',(-7.11477178379803,-1.29390043969062,
0.688772464510923));
#16267=CARTESIAN_POINT('Ctrl Pts',(-7.14099531898546,-1.06827933366594,
1.11261538880818));
#16268=CARTESIAN_POINT('Ctrl Pts',(-7.16721885417289,-0.614237919779222,
1.41486003607089));
#16269=CARTESIAN_POINT('Ctrl Pts',(-7.19344238936032,-0.136158112004879,
1.45946419653017));
#16270=CARTESIAN_POINT('Ctrl Pts',(-7.21966592454776,0.341921695769462,
1.50406835698944));
#16271=CARTESIAN_POINT('Ctrl Pts',(-7.24588945973518,0.844039897431429,
1.29103203064527));
#16272=CARTESIAN_POINT('Ctrl Pts',(-7.27211299492261,1.14416757992326,0.916230695246649));
#16273=CARTESIAN_POINT('Ctrl Pts',(-7.29833653011004,1.44429526241508,0.541429359848023));
#16274=CARTESIAN_POINT('Ctrl Pts',(-7.32456006529747,1.54243242573677,0.00486301539493375));
#16275=CARTESIAN_POINT('Ctrl Pts',(-7.3507836004849,1.39441016989669,-0.45189562140554));
#16276=CARTESIAN_POINT('Ctrl Pts',(-7.37700713567233,1.2463879140566,-0.908654258206013));
#16277=CARTESIAN_POINT('Ctrl Pts',(-7.40323067085976,0.85220623905475,-1.28560518735387));
#16278=CARTESIAN_POINT('Ctrl Pts',(-7.42945420604719,0.389290336756425,
-1.41314406620906));
#16279=CARTESIAN_POINT('Ctrl Pts',(-7.45567774123462,-0.0736255655419018,
-1.54068294506426));
#16280=CARTESIAN_POINT('Ctrl Pts',(-7.48190127642205,-0.605275695136702,
-1.41880977362678));
#16281=CARTESIAN_POINT('Ctrl Pts',(-7.50812481160948,-0.966316133086186,
-1.10223707789867));
#16282=CARTESIAN_POINT('Ctrl Pts',(-7.53069819245869,-1.27710196915086,
-0.829729348637408));
#16283=CARTESIAN_POINT('Ctrl Pts',(-7.55327157330789,-1.46146819732044,
-0.412951752401925));
#16284=CARTESIAN_POINT('Ctrl Pts',(-7.57584495415709,-1.46476825295553,
0.00111815863164652));
#16285=CARTESIAN_POINT('Ctrl Pts',(-7.64715504584291,-1.46461339238561,
0.00160511507277402));
#16286=CARTESIAN_POINT('Ctrl Pts',(-7.62448962685375,-1.46127603772873,
-0.413880441134546));
#16287=CARTESIAN_POINT('Ctrl Pts',(-7.60182420786459,-1.27550058420875,
-0.833058365384661));
#16288=CARTESIAN_POINT('Ctrl Pts',(-7.57915878887542,-0.962575882149317,
-1.10580548228527));
#16289=CARTESIAN_POINT('Ctrl Pts',(-7.55293525368799,-0.600526897332635,
-1.4213696296206));
#16290=CARTESIAN_POINT('Ctrl Pts',(-7.52671171850056,-0.0682743009747437,
-1.54091962399734));
#16291=CARTESIAN_POINT('Ctrl Pts',(-7.50048818331313,0.394239944793519,
-1.41166012590963));
#16292=CARTESIAN_POINT('Ctrl Pts',(-7.4742646481257,0.856754190561782,-1.28240062782193));
#16293=CARTESIAN_POINT('Ctrl Pts',(-7.44804111293827,1.24953008574042,-0.904331637269769));
#16294=CARTESIAN_POINT('Ctrl Pts',(-7.42181757775084,1.3959439261357,-0.447121059668684));
#16295=CARTESIAN_POINT('Ctrl Pts',(-7.39559404256341,1.54235776653098,0.0100895179324009));
#16296=CARTESIAN_POINT('Ctrl Pts',(-7.36937050737598,1.4424095521429,0.546441682582412));
#16297=CARTESIAN_POINT('Ctrl Pts',(-7.34314697218855,1.14099511095998,0.92023014033236));
#16298=CARTESIAN_POINT('Ctrl Pts',(-7.31692343700112,0.839580669777048,
1.29401859808231));
#16299=CARTESIAN_POINT('Ctrl Pts',(-7.29069990181369,0.336700001799267,
1.50524334893219));
#16300=CARTESIAN_POINT('Ctrl Pts',(-7.26447636662626,-0.141228388432861,
1.45896449548521));
#16301=CARTESIAN_POINT('Ctrl Pts',(-7.23825283143883,-0.619156778664989,
1.41268564203822));
#16302=CARTESIAN_POINT('Ctrl Pts',(-7.2120292962514,-1.07213289115146,1.10890318429437));
#16303=CARTESIAN_POINT('Ctrl Pts',(-7.18580576106397,-1.29627871914772,
0.684288464279752));
#16304=CARTESIAN_POINT('Ctrl Pts',(-7.17292218932362,-1.40640112768838,
0.47567607970926));
#16305=CARTESIAN_POINT('Ctrl Pts',(-7.16003861758326,-1.4612899065398,0.23789795580647));
#16306=CARTESIAN_POINT('Ctrl Pts',(-7.14715504584291,-1.46119347856455,
7.51979904560513E-5));
#16307=CARTESIAN_POINT('Origin',(-4.675,0.,0.));
#16308=CARTESIAN_POINT('',(-6.57584495415709,-1.46465303558881,-0.00106776041762152));
#16309=CARTESIAN_POINT('',(-6.64715504584291,-1.46460737782915,-0.00108331802881356));
#16310=CARTESIAN_POINT('',(-4.675,-1.4635,-1.79227059055215E-16));
#16311=CARTESIAN_POINT('Ctrl Pts',(-6.57584495415709,-1.46465303558881,
-0.00106776041762152));
#16312=CARTESIAN_POINT('Ctrl Pts',(-6.59814601957949,-1.46128671630142,
0.408115865061178));
#16313=CARTESIAN_POINT('Ctrl Pts',(-6.62044708500189,-1.28183534078177,
0.819889960702766));
#16314=CARTESIAN_POINT('Ctrl Pts',(-6.64274815042429,-0.977572876370026,
1.09221589872146));
#16315=CARTESIAN_POINT('Ctrl Pts',(-6.66897168561172,-0.619794568895003,
1.4124404567334));
#16316=CARTESIAN_POINT('Ctrl Pts',(-6.69519522079915,-0.089438661254516,
1.53984858630397));
#16317=CARTESIAN_POINT('Ctrl Pts',(-6.72141875598658,0.374758584894471,
1.41708857457618));
#16318=CARTESIAN_POINT('Ctrl Pts',(-6.74764229117401,0.838955831043458,
1.2943285628484));
#16319=CARTESIAN_POINT('Ctrl Pts',(-6.77386582636144,1.23699441570095,0.921400409822262));
#16320=CARTESIAN_POINT('Ctrl Pts',(-6.80008936154887,1.38969975267005,0.466174873903159));
#16321=CARTESIAN_POINT('Ctrl Pts',(-6.8263128967363,1.54240508963915,0.0109493379840572));
#16322=CARTESIAN_POINT('Ctrl Pts',(-6.85253643192373,1.44977717891987,-0.526573580828016));
#16323=CARTESIAN_POINT('Ctrl Pts',(-6.87875996711116,1.1535120245824,-0.904430536719963));
#16324=CARTESIAN_POINT('Ctrl Pts',(-6.90498350229859,0.857246870244925,
-1.28228749261191));
#16325=CARTESIAN_POINT('Ctrl Pts',(-6.93120703748602,0.357344472289264,
-1.50047848558374));
#16326=CARTESIAN_POINT('Ctrl Pts',(-6.95743057267345,-0.121167596084266,
-1.46078787938538));
#16327=CARTESIAN_POINT('Ctrl Pts',(-6.98365410786088,-0.599679664457794,
-1.42109727318701));
#16328=CARTESIAN_POINT('Ctrl Pts',(-7.00987764304832,-1.05680140324919,
-1.12352506781847));
#16329=CARTESIAN_POINT('Ctrl Pts',(-7.03610117823574,-1.28676187356357,
-0.702018364468302));
#16330=CARTESIAN_POINT('Ctrl Pts',(-7.04934910354286,-1.40293610836982,
-0.489076467713321));
#16331=CARTESIAN_POINT('Ctrl Pts',(-7.06259702884998,-1.46113443639422,
-0.244504113221373));
#16332=CARTESIAN_POINT('Ctrl Pts',(-7.07584495415709,-1.46119452374026,
4.09982538755738E-5));
#16333=CARTESIAN_POINT('Ctrl Pts',(-7.14715504584291,-1.46119347856455,
7.51979904560513E-5));
#16334=CARTESIAN_POINT('Ctrl Pts',(-7.13381508239583,-1.46109363469431,
-0.246172268169273));
#16335=CARTESIAN_POINT('Ctrl Pts',(-7.12047511894875,-1.40204395744491,
-0.492467586504148));
#16336=CARTESIAN_POINT('Ctrl Pts',(-7.10713515550167,-1.28432021657575,
-0.706483940746703));
#16337=CARTESIAN_POINT('Ctrl Pts',(-7.08091162031424,-1.05290034250147,
-1.12719464347314));
#16338=CARTESIAN_POINT('Ctrl Pts',(-7.05468808512682,-0.594745050846875,
-1.42316906664063));
#16339=CARTESIAN_POINT('Ctrl Pts',(-7.02846454993939,-0.11609725943412,
-1.4611967717883));
#16340=CARTESIAN_POINT('Ctrl Pts',(-7.00224101475196,0.362550531978637,
-1.49922447693597));
#16341=CARTESIAN_POINT('Ctrl Pts',(-6.97601747956452,0.861690823149552,
-1.27930546406382));
#16342=CARTESIAN_POINT('Ctrl Pts',(-6.94979394437709,1.15664263658477,-0.900424064368463));
#16343=CARTESIAN_POINT('Ctrl Pts',(-6.92357040918966,1.45159445001998,-0.521542664673106));
#16344=CARTESIAN_POINT('Ctrl Pts',(-6.89734687400224,1.5423577857195,0.0163011218454547));
#16345=CARTESIAN_POINT('Ctrl Pts',(-6.87112333881481,1.38807410635408,0.470994697121732));
#16346=CARTESIAN_POINT('Ctrl Pts',(-6.84489980362738,1.23379042698866,0.925688272398011));
#16347=CARTESIAN_POINT('Ctrl Pts',(-6.81867626843994,0.834459732558295,
1.297231636432));
#16348=CARTESIAN_POINT('Ctrl Pts',(-6.79245273325251,0.369839221643031,
1.41837991588424));
#16349=CARTESIAN_POINT('Ctrl Pts',(-6.76622919806508,-0.0947812892722306,
1.53952819533647));
#16350=CARTESIAN_POINT('Ctrl Pts',(-6.74000566287766,-0.624691616672391,
1.41028139020694));
#16351=CARTESIAN_POINT('Ctrl Pts',(-6.71378212769023,-0.981356587747756,
1.08881755089876));
#16352=CARTESIAN_POINT('Ctrl Pts',(-6.69157310040779,-1.28342044056879,
0.816565959857179));
#16353=CARTESIAN_POINT('Ctrl Pts',(-6.66936407312535,-1.46122233297314,
0.406444783164266));
#16354=CARTESIAN_POINT('Ctrl Pts',(-6.64715504584291,-1.46460737782915,
-0.00108331802881356));
#16355=CARTESIAN_POINT('Origin',(-4.675,0.,0.));
#16356=CARTESIAN_POINT('',(-6.0758449541571,-1.46387947857031,0.00124550601554009));
#16357=CARTESIAN_POINT('',(-6.14715504584291,-1.46392911471344,0.00123902392529235));
#16358=CARTESIAN_POINT('',(-4.675,-1.4635,-1.79227059055215E-16));
#16359=CARTESIAN_POINT('Ctrl Pts',(-6.0758449541571,-1.46387947857031,0.00124550601554009));
#16360=CARTESIAN_POINT('Ctrl Pts',(-6.08124793993415,-1.46476817976019,
0.100516198434922));
#16361=CARTESIAN_POINT('Ctrl Pts',(-6.08665092571121,-1.45551439595261,
0.199622273041832));
#16362=CARTESIAN_POINT('Ctrl Pts',(-6.09205391148826,-1.43550278566529,
0.296506294697566));
#16363=CARTESIAN_POINT('Ctrl Pts',(-6.11827744667569,-1.33837590283036,
0.766735470902046));
#16364=CARTESIAN_POINT('Ctrl Pts',(-6.14450098186312,-0.987829908906021,
1.18462036689892));
#16365=CARTESIAN_POINT('Ctrl Pts',(-6.17072451705055,-0.541660829647773,
1.36205278094015));
#16366=CARTESIAN_POINT('Ctrl Pts',(-6.19694805223798,-0.095491750389521,
1.53948519498138));
#16367=CARTESIAN_POINT('Ctrl Pts',(-6.22317158742541,0.446300414202636,
1.47646512706695));
#16368=CARTESIAN_POINT('Ctrl Pts',(-6.24939512261284,0.839831405567041,
1.20136066058004));
#16369=CARTESIAN_POINT('Ctrl Pts',(-6.27561865780027,1.23336239693144,0.926256194093134));
#16370=CARTESIAN_POINT('Ctrl Pts',(-6.3018421929877,1.47863221506809,0.439067329033746));
#16371=CARTESIAN_POINT('Ctrl Pts',(-6.32806572817513,1.46523422670663,-0.0409010089182408));
#16372=CARTESIAN_POINT('Ctrl Pts',(-6.35428926336256,1.45183623834517,-0.520869346870228));
#16373=CARTESIAN_POINT('Ctrl Pts',(-6.38051279854999,1.17977044348559,-0.993617157714814));
#16374=CARTESIAN_POINT('Ctrl Pts',(-6.40673633373742,0.77150551348923,-1.24634003584463));
#16375=CARTESIAN_POINT('Ctrl Pts',(-6.43295986892485,0.363240583492865,
-1.49906291397444));
#16376=CARTESIAN_POINT('Ctrl Pts',(-6.45918340411228,-0.181223481640291,
-1.53176085938949));
#16377=CARTESIAN_POINT('Ctrl Pts',(-6.48540693929971,-0.616799689488656,
-1.32971513666244));
#16378=CARTESIAN_POINT('Ctrl Pts',(-6.51163047448714,-1.05237589733702,
-1.1276694139354));
#16379=CARTESIAN_POINT('Ctrl Pts',(-6.53785400967457,-1.3790642479006,-0.690880023066263));
#16380=CARTESIAN_POINT('Ctrl Pts',(-6.564077544862,-1.4498080695276,-0.215964834405035));
#16381=CARTESIAN_POINT('Ctrl Pts',(-6.56800001462703,-1.46038980457634,
-0.14492786493607));
#16382=CARTESIAN_POINT('Ctrl Pts',(-6.57192248439206,-1.46524512773213,
-0.0730378824223954));
#16383=CARTESIAN_POINT('Ctrl Pts',(-6.57584495415709,-1.46465303558881,
-0.00106776041762152));
#16384=CARTESIAN_POINT('Ctrl Pts',(-6.64715504584291,-1.46460737782915,
-0.00108331802881356));
#16385=CARTESIAN_POINT('Ctrl Pts',(-6.64314053793791,-1.46521925916732,
-0.0747481734472876));
#16386=CARTESIAN_POINT('Ctrl Pts',(-6.63912603003292,-1.4601322017168,-0.148328302081877));
#16387=CARTESIAN_POINT('Ctrl Pts',(-6.63511152212793,-1.44904998055347,
-0.220994103));
#16388=CARTESIAN_POINT('Ctrl Pts',(-6.6088879869405,-1.37665878753324,-0.695661044103762));
#16389=CARTESIAN_POINT('Ctrl Pts',(-6.58266445175308,-1.04845678674222,
-1.13131405282446));
#16390=CARTESIAN_POINT('Ctrl Pts',(-6.55644091656565,-0.612182151683762,
-1.3318471614882));
#16391=CARTESIAN_POINT('Ctrl Pts',(-6.53021738137822,-0.175907516625305,
-1.53238027015193));
#16392=CARTESIAN_POINT('Ctrl Pts',(-6.50399384619078,0.368439752700586,
-1.4977934787587));
#16393=CARTESIAN_POINT('Ctrl Pts',(-6.47777031100335,0.775825313355198,
-1.24365558141487));
#16394=CARTESIAN_POINT('Ctrl Pts',(-6.45154677581592,1.18321087400981,-0.989517684071032));
#16395=CARTESIAN_POINT('Ctrl Pts',(-6.4253232406285,1.45363472599314,-0.515828680776595));
#16396=CARTESIAN_POINT('Ctrl Pts',(-6.39909970544107,1.46536726876187,-0.0358167504139053));
#16397=CARTESIAN_POINT('Ctrl Pts',(-6.37287617025364,1.4770998115306,0.444195179948787));
#16398=CARTESIAN_POINT('Ctrl Pts',(-6.3466526350662,1.23014104508472,0.930530037379732));
#16399=CARTESIAN_POINT('Ctrl Pts',(-6.32042909987877,0.835657892526212,
1.20426737561557));
#16400=CARTESIAN_POINT('Ctrl Pts',(-6.29420556469134,0.441174739967705,
1.47800471385141));
#16401=CARTESIAN_POINT('Ctrl Pts',(-6.26798202950391,-0.100832798703432,
1.53914453289215));
#16402=CARTESIAN_POINT('Ctrl Pts',(-6.24175849431648,-0.546383526501062,
1.36016510324213));
#16403=CARTESIAN_POINT('Ctrl Pts',(-6.21553495912905,-0.991934254298693,
1.18118567359212));
#16404=CARTESIAN_POINT('Ctrl Pts',(-6.18931142394163,-1.34102817122282,
0.762086995251349));
#16405=CARTESIAN_POINT('Ctrl Pts',(-6.1630878887542,-1.43652288894978,0.291523661031353));
#16406=CARTESIAN_POINT('Ctrl Pts',(-6.1577769411171,-1.45586305196907,0.19622235210727));
#16407=CARTESIAN_POINT('Ctrl Pts',(-6.15246599348001,-1.46480139245222,
0.098810128720388));
#16408=CARTESIAN_POINT('Ctrl Pts',(-6.14715504584291,-1.46392911471344,
0.00123902392529235));
#16409=CARTESIAN_POINT('Origin',(-4.675,0.,0.));
#16410=CARTESIAN_POINT('',(-5.57584495415709,-1.46133774784058,-0.000461094909492699));
#16411=CARTESIAN_POINT('',(-5.64715504584291,-1.46132187471162,-0.000435916869068641));
#16412=CARTESIAN_POINT('',(-4.675,-1.4635,-1.79227059055215E-16));
#16413=CARTESIAN_POINT('Ctrl Pts',(-5.57584495415709,-1.46133774784058,
-0.000461094909492699));
#16414=CARTESIAN_POINT('Ctrl Pts',(-5.59057339547623,-1.46055568691757,
0.271345601813848));
#16415=CARTESIAN_POINT('Ctrl Pts',(-5.60530183679537,-1.3877585012757,0.543541520393028));
#16416=CARTESIAN_POINT('Ctrl Pts',(-5.62003027811452,-1.24559580904415,
0.772706484360848));
#16417=CARTESIAN_POINT('Ctrl Pts',(-5.64625381330195,-0.992479523261131,
1.1807276297163));
#16418=CARTESIAN_POINT('Ctrl Pts',(-5.67247734848938,-0.519469702169433,
1.45233762200152));
#16419=CARTESIAN_POINT('Ctrl Pts',(-5.69870088367681,-0.0394886755002852,
1.46527296946528));
#16420=CARTESIAN_POINT('Ctrl Pts',(-5.72492441886424,0.440492351168856,
1.47820831692904));
#16421=CARTESIAN_POINT('Ctrl Pts',(-5.75114795405167,0.927444583415449,
1.23246901957134));
#16422=CARTESIAN_POINT('Ctrl Pts',(-5.7773714892391,1.2021696047976,0.838673042208838));
#16423=CARTESIAN_POINT('Ctrl Pts',(-5.80359502442652,1.47689462617977,0.444877064846331));
#16424=CARTESIAN_POINT('Ctrl Pts',(-5.82981855961395,1.53939243669748,-0.0969755925209766));
#16425=CARTESIAN_POINT('Ctrl Pts',(-5.85604209480139,1.36153004874535,-0.542973440251071));
#16426=CARTESIAN_POINT('Ctrl Pts',(-5.88226562998882,1.18366766079323,-0.988971287981157));
#16427=CARTESIAN_POINT('Ctrl Pts',(-5.90848916517625,0.765445074371262,
-1.33911432607403));
#16428=CARTESIAN_POINT('Ctrl Pts',(-5.93471270036368,0.295122497836863,
-1.4357879168145));
#16429=CARTESIAN_POINT('Ctrl Pts',(-5.96093623555111,-0.175200078697542,
-1.53246150755497));
#16430=CARTESIAN_POINT('Ctrl Pts',(-5.98715977073854,-0.697622645344382,
-1.37566565094302));
#16431=CARTESIAN_POINT('Ctrl Pts',(-6.01338330592597,-1.03698004279505,
-1.03598099443101));
#16432=CARTESIAN_POINT('Ctrl Pts',(-6.03420385533634,-1.30641768386431,
-0.766283521367007));
#16433=CARTESIAN_POINT('Ctrl Pts',(-6.05502440474672,-1.46045484489581,
-0.381296747805956));
#16434=CARTESIAN_POINT('Ctrl Pts',(-6.0758449541571,-1.46387947857031,0.00124550601554009));
#16435=CARTESIAN_POINT('Ctrl Pts',(-6.14715504584291,-1.46392911471344,
0.00123902392529235));
#16436=CARTESIAN_POINT('Ctrl Pts',(-6.12624245829258,-1.46049440101887,
-0.382960635125922));
#16437=CARTESIAN_POINT('Ctrl Pts',(-6.10532987074223,-1.3049461447426,-0.769623748906194));
#16438=CARTESIAN_POINT('Ctrl Pts',(-6.0844172831919,-1.03337916355809,-1.03957277506268));
#16439=CARTESIAN_POINT('Ctrl Pts',(-6.05819374800447,-0.692845201909629,
-1.37807788683748));
#16440=CARTESIAN_POINT('Ctrl Pts',(-6.03197021281705,-0.169881760082907,
-1.53306012028788));
#16441=CARTESIAN_POINT('Ctrl Pts',(-6.00574667762961,0.300102532701756,
-1.4347552146932));
#16442=CARTESIAN_POINT('Ctrl Pts',(-5.97952314244219,0.770086825486424,
-1.33645030909852));
#16443=CARTESIAN_POINT('Ctrl Pts',(-5.95329960725475,1.18709196922903,-0.984858264458742));
#16444=CARTESIAN_POINT('Ctrl Pts',(-5.92707607206732,1.36340577873993,-0.538245981610891));
#16445=CARTESIAN_POINT('Ctrl Pts',(-5.90085253687989,1.53971958825083,-0.091633698763043));
#16446=CARTESIAN_POINT('Ctrl Pts',(-5.87462900169247,1.47534206353002,0.449998822292882));
#16447=CARTESIAN_POINT('Ctrl Pts',(-5.84840546650504,1.19925233388025,0.842839185985495));
#16448=CARTESIAN_POINT('Ctrl Pts',(-5.8221819313176,0.923162604230478,1.23567954967811));
#16449=CARTESIAN_POINT('Ctrl Pts',(-5.79595839613017,0.435360669651733,
1.47972775600741));
#16450=CARTESIAN_POINT('Ctrl Pts',(-5.76973486094274,-0.0445725656008746,
1.46512707331867));
#16451=CARTESIAN_POINT('Ctrl Pts',(-5.74351132575531,-0.524505800853484,
1.45052639062993));
#16452=CARTESIAN_POINT('Ctrl Pts',(-5.71728779056788,-0.996570336779956,
1.17727681892315));
#16453=CARTESIAN_POINT('Ctrl Pts',(-5.69106425538045,-1.24826935756838,
0.768379896395325));
#16454=CARTESIAN_POINT('Ctrl Pts',(-5.67642785220127,-1.38875264182939,
0.540158179755382));
#16455=CARTESIAN_POINT('Ctrl Pts',(-5.66179144902209,-1.46058761064619,
0.269679569506198));
#16456=CARTESIAN_POINT('Ctrl Pts',(-5.64715504584291,-1.46132187471162,
-0.000435916869068641));
#16457=CARTESIAN_POINT('Origin',(-4.675,0.,0.));
#16458=CARTESIAN_POINT('',(-5.07584495415709,-1.46540112296262,-0.000672431366979809));
#16459=CARTESIAN_POINT('',(-5.14715504584291,-1.46536904737311,-0.000697413730935374));
#16460=CARTESIAN_POINT('',(-4.675,-1.4635,-1.79227059055215E-16));
#16461=CARTESIAN_POINT('Ctrl Pts',(-5.07584495415709,-1.46540112296262,
-0.000672431366979809));
#16462=CARTESIAN_POINT('Ctrl Pts',(-5.09989885101832,-1.46285813334839,
0.440080771362054));
#16463=CARTESIAN_POINT('Ctrl Pts',(-5.12395274787955,-1.25017446102815,
0.882964196354943));
#16464=CARTESIAN_POINT('Ctrl Pts',(-5.14800664474077,-0.903318012573032,
1.1543832979786));
#16465=CARTESIAN_POINT('Ctrl Pts',(-5.1742301799282,-0.525175446587734,
1.45028414111565));
#16466=CARTESIAN_POINT('Ctrl Pts',(-5.20045371511563,0.0124360176124621,
1.54239381648727));
#16467=CARTESIAN_POINT('Ctrl Pts',(-5.22667725030307,0.467514036020018,
1.38924974594796));
#16468=CARTESIAN_POINT('Ctrl Pts',(-5.25290078549049,0.92259205442756,1.23610567540865));
#16469=CARTESIAN_POINT('Ctrl Pts',(-5.27912432067793,1.29513662704247,0.837707858958433));
#16470=CARTESIAN_POINT('Ctrl Pts',(-5.30534785586535,1.41744920979827,0.373392512153981));
#16471=CARTESIAN_POINT('Ctrl Pts',(-5.33157139105279,1.53976179255407,-0.0909228346504821));
#16472=CARTESIAN_POINT('Ctrl Pts',(-5.35779492624021,1.41184238545076,-0.621155711809182));
#16473=CARTESIAN_POINT('Ctrl Pts',(-5.38401846142764,1.09127308713034,-0.978625198834701));
#16474=CARTESIAN_POINT('Ctrl Pts',(-5.41024199661507,0.770703788809914,
-1.33609468586022));
#16475=CARTESIAN_POINT('Ctrl Pts',(-5.43646553180251,0.257484599272379,
-1.52080078275256));
#16476=CARTESIAN_POINT('Ctrl Pts',(-5.46268906698994,-0.2173621630815,-1.44959922756557));
#16477=CARTESIAN_POINT('Ctrl Pts',(-5.48891260217737,-0.692208925435379,
-1.37839767237858));
#16478=CARTESIAN_POINT('Ctrl Pts',(-5.5151361373648,-1.1286832606056,-1.05128846511227));
#16479=CARTESIAN_POINT('Ctrl Pts',(-5.54135967255222,-1.33030905295355,
-0.61551771226628));
#16480=CARTESIAN_POINT('Ctrl Pts',(-5.55285476642051,-1.41869177453332,
-0.424497482796187));
#16481=CARTESIAN_POINT('Ctrl Pts',(-5.5643498602888,-1.46194812225331,-0.212597832610591));
#16482=CARTESIAN_POINT('Ctrl Pts',(-5.57584495415709,-1.46133774784058,
-0.000461094909492699));
#16483=CARTESIAN_POINT('Ctrl Pts',(-5.64715504584291,-1.46132187471162,
-0.000435916869068641));
#16484=CARTESIAN_POINT('Ctrl Pts',(-5.63556791383466,-1.46190316606789,
-0.214276965095653));
#16485=CARTESIAN_POINT('Ctrl Pts',(-5.62398078182641,-1.41792323597311,
-0.427890431283265));
#16486=CARTESIAN_POINT('Ctrl Pts',(-5.61239364981816,-1.32816529847952,
-0.620129820373049));
#16487=CARTESIAN_POINT('Ctrl Pts',(-5.58617011463073,-1.12502871295185,
-1.05519834126473));
#16488=CARTESIAN_POINT('Ctrl Pts',(-5.5599465794433,-0.687422036246132,
-1.38079110969925));
#16489=CARTESIAN_POINT('Ctrl Pts',(-5.53372304425587,-0.212331100229578,
-1.45034463428116));
#16490=CARTESIAN_POINT('Ctrl Pts',(-5.50749950906844,0.262759835786984,
-1.51989815886308));
#16491=CARTESIAN_POINT('Ctrl Pts',(-5.48127597388101,0.775335031114387,
-1.33341243959239));
#16492=CARTESIAN_POINT('Ctrl Pts',(-5.45505243869358,1.09466205718752,-0.974832824031823));
#16493=CARTESIAN_POINT('Ctrl Pts',(-5.42882890350615,1.41398908326066,-0.616253208471257));
#16494=CARTESIAN_POINT('Ctrl Pts',(-5.40260536831872,1.54006794007953,-0.0855796966208218));
#16495=CARTESIAN_POINT('Ctrl Pts',(-5.37638183313129,1.41614504088793,0.378308442182405));
#16496=CARTESIAN_POINT('Ctrl Pts',(-5.35015829794386,1.29222214169632,0.84219658098563));
#16497=CARTESIAN_POINT('Ctrl Pts',(-5.32393476275643,0.918297486494231,
1.23929934674164));
#16498=CARTESIAN_POINT('Ctrl Pts',(-5.297711227569,0.462690854646623,1.39086348262469));
#16499=CARTESIAN_POINT('Ctrl Pts',(-5.27148769238157,0.00708422279901214,
1.54242761850773));
#16500=CARTESIAN_POINT('Ctrl Pts',(-5.24526415719414,-0.530204385694121,
1.4484531245178));
#16501=CARTESIAN_POINT('Ctrl Pts',(-5.21904062200671,-0.907317958243424,
1.15124201491802));
#16502=CARTESIAN_POINT('Ctrl Pts',(-5.19507876328544,-1.25190697275698,
0.879664191115139));
#16503=CARTESIAN_POINT('Ctrl Pts',(-5.17111690456418,-1.46275843823164,
0.438394712888951));
#16504=CARTESIAN_POINT('Ctrl Pts',(-5.14715504584291,-1.46536904737311,
-0.000697413730935374));
#16505=CARTESIAN_POINT('Origin',(-4.675,0.,0.));
#16506=CARTESIAN_POINT('',(-4.57584495415709,-1.46294334847319,0.0012518377109378));
#16507=CARTESIAN_POINT('',(-4.64715504584291,-1.46299075660548,0.00125694264917424));
#16508=CARTESIAN_POINT('',(-4.675,-1.4635,-1.79227059055215E-16));
#16509=CARTESIAN_POINT('Ctrl Pts',(-4.57584495415709,-1.46294334847319,
0.0012518377109378));
#16510=CARTESIAN_POINT('Ctrl Pts',(-4.58300077137298,-1.4640569200179,0.132943452584338));
#16511=CARTESIAN_POINT('Ctrl Pts',(-4.59015658858886,-1.44770968903095,
0.26436354906558));
#16512=CARTESIAN_POINT('Ctrl Pts',(-4.59731240580474,-1.412790863166,0.390648444827308));
#16513=CARTESIAN_POINT('Ctrl Pts',(-4.62353594099217,-1.28482573617244,
0.853437852066254));
#16514=CARTESIAN_POINT('Ctrl Pts',(-4.6497594761796,-0.907450989065814,
1.24726342130028));
#16515=CARTESIAN_POINT('Ctrl Pts',(-4.67598301136703,-0.450539437904677,
1.39484710466189));
#16516=CARTESIAN_POINT('Ctrl Pts',(-4.70220654655446,0.00637211325646751,
1.5424307880235));
#16517=CARTESIAN_POINT('Ctrl Pts',(-4.72843008174189,0.542820468472122,
1.44377258551269));
#16518=CARTESIAN_POINT('Ctrl Pts',(-4.75465361692932,0.917326849766136,
1.14328285266129));
#16519=CARTESIAN_POINT('Ctrl Pts',(-4.78087715211675,1.29183323106015,0.8427931198099));
#16520=CARTESIAN_POINT('Ctrl Pts',(-4.80710068730418,1.50439763843252,0.340471856617928));
#16521=CARTESIAN_POINT('Ctrl Pts',(-4.83332422249161,1.45933557059906,-0.13756424999078));
#16522=CARTESIAN_POINT('Ctrl Pts',(-4.85954775767904,1.4142735027656,-0.61560035659948));
#16523=CARTESIAN_POINT('Ctrl Pts',(-4.88577129286647,1.1115849597263,-1.06935130662492));
#16524=CARTESIAN_POINT('Ctrl Pts',(-4.9119948280539,0.687523242977742,-1.29456402732985));
#16525=CARTESIAN_POINT('Ctrl Pts',(-4.93821836324133,0.263461526229175,
-1.51977674803479));
#16526=CARTESIAN_POINT('Ctrl Pts',(-4.96444189842876,-0.281973364228664,
-1.51645123941922));
#16527=CARTESIAN_POINT('Ctrl Pts',(-4.99066543361619,-0.703257419359688,
-1.28608445780473));
#16528=CARTESIAN_POINT('Ctrl Pts',(-5.01688896880362,-1.12454147449071,
-1.05571767619023));
#16529=CARTESIAN_POINT('Ctrl Pts',(-5.04311250399105,-1.42167469429492,
-0.598309621576813));
#16530=CARTESIAN_POINT('Ctrl Pts',(-5.06933603917848,-1.46090447031182,
-0.119759588818864));
#16531=CARTESIAN_POINT('Ctrl Pts',(-5.07150567750469,-1.46415019690689,
-0.0801661287969205));
#16532=CARTESIAN_POINT('Ctrl Pts',(-5.07367531583089,-1.46563049817621,
-0.0404279456836342));
#16533=CARTESIAN_POINT('Ctrl Pts',(-5.07584495415709,-1.46540112296262,
-0.000672431366979809));
#16534=CARTESIAN_POINT('Ctrl Pts',(-5.14715504584291,-1.46536904737311,
-0.000697413730935374));
#16535=CARTESIAN_POINT('Ctrl Pts',(-5.14489336937675,-1.465615453686,-0.0421417916819987));
#16536=CARTESIAN_POINT('Ctrl Pts',(-5.14263169291058,-1.46400668068721,
-0.0835667720099182));
#16537=CARTESIAN_POINT('Ctrl Pts',(-5.14037001644442,-1.46048008062653,
-0.12482783486786));
#16538=CARTESIAN_POINT('Ctrl Pts',(-5.11414648125699,-1.41959009385488,
-0.603238849844358));
#16539=CARTESIAN_POINT('Ctrl Pts',(-5.08792294606956,-1.12087158370608,
-1.05961315458773));
#16540=CARTESIAN_POINT('Ctrl Pts',(-5.06169941088213,-0.698790766895836,
-1.28851679009923));
#16541=CARTESIAN_POINT('Ctrl Pts',(-5.0354758756947,-0.276709950085593,
-1.51742042561072));
#16542=CARTESIAN_POINT('Ctrl Pts',(-5.00925234050727,0.268733173386092,
-1.51885339189034));
#16543=CARTESIAN_POINT('Ctrl Pts',(-4.98302880531984,0.692010888444511,
-1.29217064838177));
#16544=CARTESIAN_POINT('Ctrl Pts',(-4.95680527013241,1.11528860350292,-1.0654879048732));
#16545=CARTESIAN_POINT('Ctrl Pts',(-4.93058173494498,1.41640091014807,-0.610689451576441));
#16546=CARTESIAN_POINT('Ctrl Pts',(-4.90435819975755,1.45980403956193,-0.132499888090858));
#16547=CARTESIAN_POINT('Ctrl Pts',(-4.87813466457012,1.50320716897579,0.345689675394735));
#16548=CARTESIAN_POINT('Ctrl Pts',(-4.85191112938269,1.28890112115835,0.847270349069159));
#16549=CARTESIAN_POINT('Ctrl Pts',(-4.82568759419526,0.913354385642052,
1.146458817618));
#16550=CARTESIAN_POINT('Ctrl Pts',(-4.79946405900783,0.537807650125757,
1.44564728616683));
#16551=CARTESIAN_POINT('Ctrl Pts',(-4.7732405238204,0.00102022691060563,
1.54244354959008));
#16552=CARTESIAN_POINT('Ctrl Pts',(-4.74701698863297,-0.455376476747224,
1.39327539226482));
#16553=CARTESIAN_POINT('Ctrl Pts',(-4.72079345344554,-0.911773180405061,
1.24410723493957));
#16554=CARTESIAN_POINT('Ctrl Pts',(-4.69456991825811,-1.28777916450557,
0.848974656865799));
#16555=CARTESIAN_POINT('Ctrl Pts',(-4.66834638307068,-1.41413775285701,
0.385744047536753));
#16556=CARTESIAN_POINT('Ctrl Pts',(-4.66128260399475,-1.4481747027221,0.260964582749956));
#16557=CARTESIAN_POINT('Ctrl Pts',(-4.65421882491883,-1.46409746841424,
0.131243987789252));
#16558=CARTESIAN_POINT('Ctrl Pts',(-4.64715504584291,-1.46299075660548,
0.00125694264917424));
#16559=CARTESIAN_POINT('Origin',(-4.675,0.,0.));
#16560=CARTESIAN_POINT('',(-4.0758449541571,-1.46180176082141,-0.000890585205371164));
#16561=CARTESIAN_POINT('',(-4.14715504584291,-1.46177010110622,-0.000870981035757715));
#16562=CARTESIAN_POINT('',(-4.675,-1.4635,-1.79227059055215E-16));
#16563=CARTESIAN_POINT('Ctrl Pts',(-4.0758449541571,-1.46180176082141,-0.000890585205371164));
#16564=CARTESIAN_POINT('Ctrl Pts',(-4.09232622691506,-1.46007789690811,
0.303021445376408));
#16565=CARTESIAN_POINT('Ctrl Pts',(-4.10880749967303,-1.36752126553833,
0.607895648754888));
#16566=CARTESIAN_POINT('Ctrl Pts',(-4.125288772431,-1.19185385646752,0.853269368559352));
#16567=CARTESIAN_POINT('Ctrl Pts',(-4.15151230761843,-0.912347500938886,
1.24368620528404));
#16568=CARTESIAN_POINT('Ctrl Pts',(-4.17773584280586,-0.422435044033784,
1.48346957273887));
#16569=CARTESIAN_POINT('Ctrl Pts',(-4.20395937799329,0.0573525716842393,
1.46468252976897));
#16570=CARTESIAN_POINT('Ctrl Pts',(-4.23018291318072,0.537140187402255,
1.44589548679908));
#16571=CARTESIAN_POINT('Ctrl Pts',(-4.25640644836815,1.00680296193319,1.16853803340446));
#16572=CARTESIAN_POINT('Ctrl Pts',(-4.28262998355558,1.25492521704804,0.757460843943328));
#16573=CARTESIAN_POINT('Ctrl Pts',(-4.30885351874301,1.50304747216288,0.346383654482191));
#16574=CARTESIAN_POINT('Ctrl Pts',(-4.33507705393044,1.52962920786163,-0.198413271045462));
#16575=CARTESIAN_POINT('Ctrl Pts',(-4.36130058911787,1.32270482672636,-0.631693099413778));
#16576=CARTESIAN_POINT('Ctrl Pts',(-4.3875241243053,1.11578044559109,-1.0649729277821));
#16577=CARTESIAN_POINT('Ctrl Pts',(-4.41374765949273,0.675349947621797,
-1.38673565899107));
#16578=CARTESIAN_POINT('Ctrl Pts',(-4.43997119468016,0.199670289708311,
-1.45214186837879));
#16579=CARTESIAN_POINT('Ctrl Pts',(-4.46619472986759,-0.276009368205169,
-1.5175480777665));
#16580=CARTESIAN_POINT('Ctrl Pts',(-4.49241826505502,-0.786938186062845,
-1.32659776533294));
#16581=CARTESIAN_POINT('Ctrl Pts',(-4.51864180024245,-1.10312484155144,
-0.965245986494234));
#16582=CARTESIAN_POINT('Ctrl Pts',(-4.537709518214,-1.33303121878594,-0.702499039594554));
#16583=CARTESIAN_POINT('Ctrl Pts',(-4.55677723618554,-1.45997607478309,
-0.349659664898473));
#16584=CARTESIAN_POINT('Ctrl Pts',(-4.57584495415709,-1.46294334847319,
0.0012518377109378));
#16585=CARTESIAN_POINT('Ctrl Pts',(-4.64715504584291,-1.46299075660548,
0.00125694264917424));
#16586=CARTESIAN_POINT('Ctrl Pts',(-4.6279952897314,-1.45998891748883,-0.351319214641563));
#16587=CARTESIAN_POINT('Ctrl Pts',(-4.6088355336199,-1.33169977541796,-0.705855668385529));
#16588=CARTESIAN_POINT('Ctrl Pts',(-4.58967577750839,-1.09976899462203,
-0.969067702863716));
#16589=CARTESIAN_POINT('Ctrl Pts',(-4.56345224232096,-0.782330455433243,
-1.32932020335082));
#16590=CARTESIAN_POINT('Ctrl Pts',(-4.53722870713353,-0.27074218445331,
-1.51849656374072));
#16591=CARTESIAN_POINT('Ctrl Pts',(-4.5110051719461,0.204707647421047,-1.45144026172377));
#16592=CARTESIAN_POINT('Ctrl Pts',(-4.48478163675867,0.680157479295415,
-1.38438395970681));
#16593=CARTESIAN_POINT('Ctrl Pts',(-4.45855810157124,1.11946887206421,-1.06109499528299));
#16594=CARTESIAN_POINT('Ctrl Pts',(-4.43233456638381,1.32488862684911,-0.627099817183438));
#16595=CARTESIAN_POINT('Ctrl Pts',(-4.40611103119638,1.53030838163401,-0.193104639083896));
#16596=CARTESIAN_POINT('Ctrl Pts',(-4.37988749600895,1.50183649843503,0.351596752691371));
#16597=CARTESIAN_POINT('Ctrl Pts',(-4.35366396082152,1.25228941241289,0.761810528821953));
#16598=CARTESIAN_POINT('Ctrl Pts',(-4.32744042563408,1.00274232639075,1.17202430495254));
#16599=CARTESIAN_POINT('Ctrl Pts',(-4.30121689044665,0.532120037545447,
1.44775046543844));
#16600=CARTESIAN_POINT('Ctrl Pts',(-4.27499335525922,0.0522701433084407,
1.46487265193383));
#16601=CARTESIAN_POINT('Ctrl Pts',(-4.24876982007179,-0.427579750928559,
1.48199483842921));
#16602=CARTESIAN_POINT('Ctrl Pts',(-4.22254628488437,-0.916657250557259,
1.24051305093409));
#16603=CARTESIAN_POINT('Ctrl Pts',(-4.19632274969694,-1.19480726366955,
0.849128763468167));
#16604=CARTESIAN_POINT('Ctrl Pts',(-4.17993351507893,-1.36864598492955,
0.60452067126266));
#16605=CARTESIAN_POINT('Ctrl Pts',(-4.16354428046092,-1.46009593122817,
0.301360308131175));
#16606=CARTESIAN_POINT('Ctrl Pts',(-4.14715504584291,-1.46177010110622,
-0.000870981035757715));
#16607=CARTESIAN_POINT('Origin',(-4.675,0.,0.));
#16608=CARTESIAN_POINT('',(-3.57584495415709,-1.46578812638883,-0.00013691639962482));
#16609=CARTESIAN_POINT('',(-3.64715504584291,-1.46577995658709,-0.000166956455778383));
#16610=CARTESIAN_POINT('',(-4.675,-1.4635,-1.79227059055215E-16));
#16611=CARTESIAN_POINT('Ctrl Pts',(-3.57584495415709,-1.46578812638883,
-0.00013691639962482));
#16612=CARTESIAN_POINT('Ctrl Pts',(-3.60165168245715,-1.46514662501551,
0.472401287906723));
#16613=CARTESIAN_POINT('Ctrl Pts',(-3.6274584107572,-1.21566859845595,0.945522380027992));
#16614=CARTESIAN_POINT('Ctrl Pts',(-3.65326513905726,-0.825120157214755,
1.21151184763414));
#16615=CARTESIAN_POINT('Ctrl Pts',(-3.67948867424469,-0.428263931496958,
1.48179733606006));
#16616=CARTESIAN_POINT('Ctrl Pts',(-3.70571220943212,0.114256391201713,
1.53820636350536));
#16617=CARTESIAN_POINT('Ctrl Pts',(-3.73193574461955,0.558228775463752,
1.35534676916974));
#16618=CARTESIAN_POINT('Ctrl Pts',(-3.75815927980698,1.00220115972579,1.17248717483412));
#16619=CARTESIAN_POINT('Ctrl Pts',(-3.78438281499441,1.3476256055512,0.750358958717571));
#16620=CARTESIAN_POINT('Ctrl Pts',(-3.81060635018184,1.43901151974464,0.27898042309323));
#16621=CARTESIAN_POINT('Ctrl Pts',(-3.83682988536927,1.53039743393808,-0.192398112531104));
#16622=CARTESIAN_POINT('Ctrl Pts',(-3.8630534205567,1.36774481649956,-0.713026967663235));
#16623=CARTESIAN_POINT('Ctrl Pts',(-3.88927695574413,1.02427069729705,-1.04854841051664));
#16624=CARTESIAN_POINT('Ctrl Pts',(-3.91550049093156,0.680796578094537,
-1.38406985337005));
#16625=CARTESIAN_POINT('Ctrl Pts',(-3.94172402611899,0.156500957128029,
-1.53448388394474));
#16626=CARTESIAN_POINT('Ctrl Pts',(-3.96794756130642,-0.312607862765557,
-1.43208259350458));
#16627=CARTESIAN_POINT('Ctrl Pts',(-3.99417109649385,-0.781716682659144,
-1.32968130306442));
#16628=CARTESIAN_POINT('Ctrl Pts',(-4.02039463168128,-1.19563870147981,
-0.974464691609415));
#16629=CARTESIAN_POINT('Ctrl Pts',(-4.04661816686871,-1.36804958381406,
-0.52633123288464));
#16630=CARTESIAN_POINT('Ctrl Pts',(-4.05636042929817,-1.43210166715789,
-0.359845908647675));
#16631=CARTESIAN_POINT('Ctrl Pts',(-4.06610269172764,-1.4628207558276,-0.180536344418141));
#16632=CARTESIAN_POINT('Ctrl Pts',(-4.0758449541571,-1.46180176082141,-0.000890585205371164));
#16633=CARTESIAN_POINT('Ctrl Pts',(-4.14715504584291,-1.46177010110622,
-0.000870981035757715));
#16634=CARTESIAN_POINT('Ctrl Pts',(-4.13732074527349,-1.46277468064693,
-0.182223765862292));
#16635=CARTESIAN_POINT('Ctrl Pts',(-4.12748644470407,-1.43145498611871,
-0.363242032373778));
#16636=CARTESIAN_POINT('Ctrl Pts',(-4.11765214413464,-1.36621505532258,
-0.53107483170888));
#16637=CARTESIAN_POINT('Ctrl Pts',(-4.09142860894721,-1.19225030726744,
-0.978607351983263));
#16638=CARTESIAN_POINT('Ctrl Pts',(-4.06520507375979,-0.777098284561283,
-1.33238560509529));
#16639=CARTESIAN_POINT('Ctrl Pts',(-4.03898153857236,-0.307637000979528,
-1.43315858504627));
#16640=CARTESIAN_POINT('Ctrl Pts',(-4.01275800338493,0.16182428260222,-1.53393156499725));
#16641=CARTESIAN_POINT('Ctrl Pts',(-3.98653446819749,0.685594827059569,
-1.38169927178719));
#16642=CARTESIAN_POINT('Ctrl Pts',(-3.96031093301006,1.02790268941062,-1.04498809341299));
#16643=CARTESIAN_POINT('Ctrl Pts',(-3.93408739782263,1.37021055176168,-0.708276915038779));
#16644=CARTESIAN_POINT('Ctrl Pts',(-3.9078638626352,1.53105573200644,-0.187086851500426));
#16645=CARTESIAN_POINT('Ctrl Pts',(-3.88164032744778,1.43803480643175,0.283971741109459));
#16646=CARTESIAN_POINT('Ctrl Pts',(-3.85541679226035,1.34501388085707,0.755030333719338));
#16647=CARTESIAN_POINT('Ctrl Pts',(-3.82919325707291,0.998126849462947,
1.17595745540075));
#16648=CARTESIAN_POINT('Ctrl Pts',(-3.80296972188548,0.55352267908109,1.35727546872357));
#16649=CARTESIAN_POINT('Ctrl Pts',(-3.77674618669805,0.108918508699223,
1.53859348204638));
#16650=CARTESIAN_POINT('Ctrl Pts',(-3.75052265151062,-0.433402800670376,
1.4803023870106));
#16651=CARTESIAN_POINT('Ctrl Pts',(-3.72429911632319,-0.829318798459288,
1.20864154522129));
#16652=CARTESIAN_POINT('Ctrl Pts',(-3.6985844261631,-1.21755238862171,0.942252047187829));
#16653=CARTESIAN_POINT('Ctrl Pts',(-3.672869736003,-1.46500727958381,0.470692975234204));
#16654=CARTESIAN_POINT('Ctrl Pts',(-3.64715504584291,-1.46577995658709,
-0.000166956455778383));
#16655=CARTESIAN_POINT('Origin',(-4.675,0.,0.));
#16656=CARTESIAN_POINT('',(-3.07584495415709,-1.46212013789102,0.00104925812874614));
#16657=CARTESIAN_POINT('',(-3.14715504584291,-1.46215854801559,0.001064531573891));
#16658=CARTESIAN_POINT('',(-4.675,-1.4635,-1.79227059055215E-16));
#16659=CARTESIAN_POINT('Ctrl Pts',(-3.07584495415709,-1.46212013789102,
0.00104925812874614));
#16660=CARTESIAN_POINT('Ctrl Pts',(-3.0847536028118,-1.46323398523221,0.165233158946807));
#16661=CARTESIAN_POINT('Ctrl Pts',(-3.09366225146651,-1.43767095884633,
0.329080475627605));
#16662=CARTESIAN_POINT('Ctrl Pts',(-3.10257090012123,-1.38391209651775,
0.483085407287739));
#16663=CARTESIAN_POINT('Ctrl Pts',(-3.12879443530866,-1.22566728604764,
0.936414963874487));
#16664=CARTESIAN_POINT('Ctrl Pts',(-3.15501797049609,-0.823111043591577,
1.30446216942745));
#16665=CARTESIAN_POINT('Ctrl Pts',(-3.18124150568352,-0.357451444629033,
1.42155292093755));
#16666=CARTESIAN_POINT('Ctrl Pts',(-3.20746504087095,0.108208154333504,
1.53864367244765));
#16667=CARTESIAN_POINT('Ctrl Pts',(-3.23368857605837,0.636971109802517,
1.40477796991489));
#16668=CARTESIAN_POINT('Ctrl Pts',(-3.2599121112458,0.990818161946596,1.08021460904761));
#16669=CARTESIAN_POINT('Ctrl Pts',(-3.28613564643324,1.34466521409068,0.755651248180315));
#16670=CARTESIAN_POINT('Ctrl Pts',(-3.31235918162067,1.52359636290982,0.240390228978487));
#16671=CARTESIAN_POINT('Ctrl Pts',(-3.3385827168081,1.44706691016575,-0.233627019133847));
#16672=CARTESIAN_POINT('Ctrl Pts',(-3.36480625199553,1.37053745742168,-0.707644267246182));
#16673=CARTESIAN_POINT('Ctrl Pts',(-3.39102978718296,1.03854740311439,-1.14041774426902));
#16674=CARTESIAN_POINT('Ctrl Pts',(-3.41725332237039,0.600539931461536,
-1.33713724918636));
#16675=CARTESIAN_POINT('Ctrl Pts',(-3.44347685755782,0.162532459808684,
-1.5338567541037));
#16676=CARTESIAN_POINT('Ctrl Pts',(-3.46970039274525,-0.381492429189738,
-1.49452228691555));
#16677=CARTESIAN_POINT('Ctrl Pts',(-3.49592392793268,-0.786645427391987,
-1.23684000663439));
#16678=CARTESIAN_POINT('Ctrl Pts',(-3.52214746312011,-1.19179842559424,
-0.97915772635323));
#16679=CARTESIAN_POINT('Ctrl Pts',(-3.54837099830754,-1.45807953300032,
-0.503127632979056));
#16680=CARTESIAN_POINT('Ctrl Pts',(-3.57459453349497,-1.46562402233489,
-0.0230316115886923));
#16681=CARTESIAN_POINT('Ctrl Pts',(-3.57501134038234,-1.46574393733086,
-0.0154007819966268));
#16682=CARTESIAN_POINT('Ctrl Pts',(-3.57542814726972,-1.46579848733764,
-0.00776892522355069));
#16683=CARTESIAN_POINT('Ctrl Pts',(-3.57584495415709,-1.46578812638883,
-0.00013691639962482));
#16684=CARTESIAN_POINT('Ctrl Pts',(-3.64715504584291,-1.46577995658709,
-0.000166956455778383));
#16685=CARTESIAN_POINT('Ctrl Pts',(-3.64664620081557,-1.46579524640192,
-0.00948438292758694));
#16686=CARTESIAN_POINT('Ctrl Pts',(-3.64613735578824,-1.46571394306979,
-0.0188015356376304));
#16687=CARTESIAN_POINT('Ctrl Pts',(-3.6456285107609,-1.4655352260066,-0.0281168194302507));
#16688=CARTESIAN_POINT('Ctrl Pts',(-3.61940497557347,-1.45632496955679,
-0.508183753749672));
#16689=CARTESIAN_POINT('Ctrl Pts',(-3.59318144038604,-1.18839377044896,
-0.983287033845705));
#16690=CARTESIAN_POINT('Ctrl Pts',(-3.56695790519861,-0.782349135137309,
-1.23956197302861));
#16691=CARTESIAN_POINT('Ctrl Pts',(-3.54073437001118,-0.376304499825653,
-1.49583691221152));
#16692=CARTESIAN_POINT('Ctrl Pts',(-3.51451083482375,0.167853571689824,
-1.53328351048129));
#16693=CARTESIAN_POINT('Ctrl Pts',(-3.48828729963632,0.60517582193308,-1.33504542211986));
#16694=CARTESIAN_POINT('Ctrl Pts',(-3.46206376444889,1.04249807217633,-1.13680733375844));
#16695=CARTESIAN_POINT('Ctrl Pts',(-3.43584022926146,1.37298450114736,-0.702884558765829));
#16696=CARTESIAN_POINT('Ctrl Pts',(-3.40961669407403,1.44786876825344,-0.228604644891952));
#16697=CARTESIAN_POINT('Ctrl Pts',(-3.3833931588866,1.52275303535953,0.245675268981927));
#16698=CARTESIAN_POINT('Ctrl Pts',(-3.35716962369917,1.34203514060067,0.760312321737079));
#16699=CARTESIAN_POINT('Ctrl Pts',(-3.33094608851174,0.987064081362439,
1.08364595394706));
#16700=CARTESIAN_POINT('Ctrl Pts',(-3.30472255332431,0.632093022124202,
1.40697958615704));
#16701=CARTESIAN_POINT('Ctrl Pts',(-3.27849901813688,0.102868798406588,
1.53900979782185));
#16702=CARTESIAN_POINT('Ctrl Pts',(-3.25227548294945,-0.362381706248886,
1.42030403618362));
#16703=CARTESIAN_POINT('Ctrl Pts',(-3.22605194776202,-0.827632210904352,
1.30159827454539));
#16704=CARTESIAN_POINT('Ctrl Pts',(-3.19982841257459,-1.22890899649768,
0.932156539604121));
#16705=CARTESIAN_POINT('Ctrl Pts',(-3.17360487738716,-1.38557990166134,
0.478280656560232));
#16706=CARTESIAN_POINT('Ctrl Pts',(-3.16478826687241,-1.43825420129137,
0.325683119491518));
#16707=CARTESIAN_POINT('Ctrl Pts',(-3.15597165635766,-1.46327897253593,
0.163541394970867));
#16708=CARTESIAN_POINT('Ctrl Pts',(-3.14715504584291,-1.46215854801559,
0.001064531573891));
#16709=CARTESIAN_POINT('Origin',(-4.675,0.,0.));
#16710=CARTESIAN_POINT('',(-2.57584495415709,-1.46253100424383,-0.00117902711067597));
#16711=CARTESIAN_POINT('',(-2.64715504584291,-1.46248673610352,-0.00116876785021116));
#16712=CARTESIAN_POINT('',(-4.675,-1.4635,-1.79227059055215E-16));
#16713=CARTESIAN_POINT('Ctrl Pts',(-2.57584495415709,-1.46253100424383,
-0.00117902711067597));
#16714=CARTESIAN_POINT('Ctrl Pts',(-2.59407905835389,-1.45991564447785,
0.334631950775567));
#16715=CARTESIAN_POINT('Ctrl Pts',(-2.61231316255069,-1.34476101557545,
0.672063525348569));
#16716=CARTESIAN_POINT('Ctrl Pts',(-2.63054726674748,-1.1329090593835,0.930107455118416));
#16717=CARTESIAN_POINT('Ctrl Pts',(-2.65677080193491,-0.828232330120255,
1.30121557203982));
#16718=CARTESIAN_POINT('Ctrl Pts',(-2.68299433712235,-0.323556481759576,
1.50812619278528));
#16719=CARTESIAN_POINT('Ctrl Pts',(-2.70921787230977,0.153943264898992,
1.45769889133524));
#16720=CARTESIAN_POINT('Ctrl Pts',(-2.7354414074972,0.63144301155756,1.40727158988519));
#16721=CARTESIAN_POINT('Ctrl Pts',(-2.76166494268463,1.08176665651402,1.09950636623965));
#16722=CARTESIAN_POINT('Ctrl Pts',(-2.78788847787206,1.30220318772352,0.672942251246367));
#16723=CARTESIAN_POINT('Ctrl Pts',(-2.81411201305949,1.52263971893302,0.246378136253079));
#16724=CARTESIAN_POINT('Ctrl Pts',(-2.84033554824692,1.51318913639555,-0.298984870087951));
#16725=CARTESIAN_POINT('Ctrl Pts',(-2.86655908343435,1.27810593674146,-0.717655376634697));
#16726=CARTESIAN_POINT('Ctrl Pts',(-2.89278261862179,1.04302273708737,-1.13632588318144));
#16727=CARTESIAN_POINT('Ctrl Pts',(-2.91900615380921,0.582306920316665,
-1.4283038899339));
#16728=CARTESIAN_POINT('Ctrl Pts',(-2.94522968899664,0.103346550680954,
-1.46215723795242));
#16729=CARTESIAN_POINT('Ctrl Pts',(-2.97145322418407,-0.375613818954749,
-1.49601058597093));
#16730=CARTESIAN_POINT('Ctrl Pts',(-2.9976767593715,-0.872818741455455,
-1.2717392752555));
#16731=CARTESIAN_POINT('Ctrl Pts',(-3.02390029455893,-1.16445451346373,
-0.890297666087522));
#16732=CARTESIAN_POINT('Ctrl Pts',(-3.04121518109165,-1.35701590021474,
-0.638439244467571));
#16733=CARTESIAN_POINT('Ctrl Pts',(-3.05853006762437,-1.45995525957164,
-0.318059253537677));
#16734=CARTESIAN_POINT('Ctrl Pts',(-3.07584495415709,-1.46212013789102,
0.00104925812874614));
#16735=CARTESIAN_POINT('Ctrl Pts',(-3.14715504584291,-1.46215854801559,
0.001064531573891));
#16736=CARTESIAN_POINT('Ctrl Pts',(-3.12974812117023,-1.45994645696379,
-0.319718893924214));
#16737=CARTESIAN_POINT('Ctrl Pts',(-3.11234119649755,-1.35582063834627,
-0.641808687614994));
#16738=CARTESIAN_POINT('Ctrl Pts',(-3.09493427182487,-1.16135833267832,
-0.894332644230534));
#16739=CARTESIAN_POINT('Ctrl Pts',(-3.06871073663744,-0.868400833797661,
-1.27476003083089));
#16740=CARTESIAN_POINT('Ctrl Pts',(-3.04248720145001,-0.370420811302354,
-1.49730477288509));
#16741=CARTESIAN_POINT('Ctrl Pts',(-3.01626366626258,0.108419216308635,
-1.46178977272535));
#16742=CARTESIAN_POINT('Ctrl Pts',(-2.99004013107515,0.587259243919631,
-1.42627477256562));
#16743=CARTESIAN_POINT('Ctrl Pts',(-2.96381659588772,1.04695927664631,-1.13270003019193));
#16744=CARTESIAN_POINT('Ctrl Pts',(-2.93759306070029,1.28058832546627,-0.713216352864168));
#16745=CARTESIAN_POINT('Ctrl Pts',(-2.91136952551286,1.51421737428623,-0.293732675536404));
#16746=CARTESIAN_POINT('Ctrl Pts',(-2.88514599032543,1.52177543919947,0.25165993674544));
#16747=CARTESIAN_POINT('Ctrl Pts',(-2.858922455138,1.29986025823381,0.67745655287492));
#16748=CARTESIAN_POINT('Ctrl Pts',(-2.83269891995057,1.07794507726815,1.10325316900439));
#16749=CARTESIAN_POINT('Ctrl Pts',(-2.80647538476314,0.626556650423587,
1.40945378898151));
#16750=CARTESIAN_POINT('Ctrl Pts',(-2.78025184957571,0.14888466646931,1.45822408364331));
#16751=CARTESIAN_POINT('Ctrl Pts',(-2.75402831438828,-0.328787317484966,
1.50699437830511));
#16752=CARTESIAN_POINT('Ctrl Pts',(-2.72780477920085,-0.832742858548961,
1.29833434765159));
#16753=CARTESIAN_POINT('Ctrl Pts',(-2.70158124401342,-1.13612978259562,
0.926171131866864));
#16754=CARTESIAN_POINT('Ctrl Pts',(-2.68343917795658,-1.34602008066168,
0.668699757529504));
#16755=CARTESIAN_POINT('Ctrl Pts',(-2.66529711189975,-1.4599141899931,0.33297245835215));
#16756=CARTESIAN_POINT('Ctrl Pts',(-2.64715504584291,-1.46248673610352,
-0.00116876785021116));
#16757=CARTESIAN_POINT('Origin',(-4.675,0.,0.));
#16758=CARTESIAN_POINT('',(-2.07584495415709,-1.46567283994288,0.000450589203851749));
#16759=CARTESIAN_POINT('',(-2.14715504584291,-1.46566693596749,0.000405098676182412));
#16760=CARTESIAN_POINT('',(-4.675,-1.4635,-1.79227059055215E-16));
#16761=CARTESIAN_POINT('Ctrl Pts',(-2.07584495415709,-1.46567283994288,
0.000450589203851749));
#16762=CARTESIAN_POINT('Ctrl Pts',(-2.07718097870854,-1.46577104663176,
0.0249220526474152));
#16763=CARTESIAN_POINT('Ctrl Pts',(-2.07851700326,-1.46521215258492,0.0493888675234306));
#16764=CARTESIAN_POINT('Ctrl Pts',(-2.07985302781145,-1.46398217331303,
0.0738216850181092));
#16765=CARTESIAN_POINT('Ctrl Pts',(-2.10607656299888,-1.43984009846771,
0.553389855081013));
#16766=CARTESIAN_POINT('Ctrl Pts',(-2.13230009818631,-1.15715592121758,
1.01986020370653));
#16767=CARTESIAN_POINT('Ctrl Pts',(-2.15852363337374,-0.743301695393459,
1.26333911036547));
#16768=CARTESIAN_POINT('Ctrl Pts',(-2.18474716856117,-0.329447469569337,
1.50681801702441));
#16769=CARTESIAN_POINT('Ctrl Pts',(-2.2109707037486,0.215576804828768,1.52730548171678));
#16770=CARTESIAN_POINT('Ctrl Pts',(-2.23719423893603,0.646496882664062,
1.31553455114735));
#16771=CARTESIAN_POINT('Ctrl Pts',(-2.26341777412346,1.07741696049935,1.10376362057792));
#16772=CARTESIAN_POINT('Ctrl Pts',(-2.28964130931089,1.39423284177183,0.659734294746721));
#16773=CARTESIAN_POINT('Ctrl Pts',(-2.31586484449832,1.45429777609794,0.183346983329943));
#16774=CARTESIAN_POINT('Ctrl Pts',(-2.34208837968575,1.51436271042405,-0.293040328086842));
#16775=CARTESIAN_POINT('Ctrl Pts',(-2.36831191487318,1.31767669780378,-0.801785625089211));
#16776=CARTESIAN_POINT('Ctrl Pts',(-2.39453545006061,0.952794611848804,
-1.11389281353731));
#16777=CARTESIAN_POINT('Ctrl Pts',(-2.42075898524804,0.587912525893835,
-1.4260000019854));
#16778=CARTESIAN_POINT('Ctrl Pts',(-2.44698252043547,0.0548343666041687,
-1.54146908187924));
#16779=CARTESIAN_POINT('Ctrl Pts',(-2.4732060556229,-0.406487582422807,
-1.40831590953028));
#16780=CARTESIAN_POINT('Ctrl Pts',(-2.49942959081033,-0.867809531449795,
-1.27516273718131));
#16781=CARTESIAN_POINT('Ctrl Pts',(-2.52565312599776,-1.25737527021408,
-0.893387312589523));
#16782=CARTESIAN_POINT('Ctrl Pts',(-2.55187666118519,-1.39981933451332,
-0.434846793744943));
#16783=CARTESIAN_POINT('Ctrl Pts',(-2.55986609217582,-1.44321725983536,
-0.295144888356011));
#16784=CARTESIAN_POINT('Ctrl Pts',(-2.56785552316646,-1.46367694682157,
-0.148317521262214));
#16785=CARTESIAN_POINT('Ctrl Pts',(-2.57584495415709,-1.46253100424383,
-0.00117902711067597));
#16786=CARTESIAN_POINT('Ctrl Pts',(-2.64715504584291,-1.46248673610352,
-0.00116876785021116));
#16787=CARTESIAN_POINT('Ctrl Pts',(-2.63907357671231,-1.46363268893565,
-0.150013557432222));
#16788=CARTESIAN_POINT('Ctrl Pts',(-2.63099210758172,-1.44268911331045,
-0.298543622686762));
#16789=CARTESIAN_POINT('Ctrl Pts',(-2.62291063845113,-1.39830137570459,
-0.439701606098301));
#16790=CARTESIAN_POINT('Ctrl Pts',(-2.5966871032637,-1.25426773773756,-0.897744727362739));
#16791=CARTESIAN_POINT('Ctrl Pts',(-2.57046356807627,-0.863382154774179,
-1.27816456897568));
#16792=CARTESIAN_POINT('Ctrl Pts',(-2.54424003288884,-0.401599883091991,
-1.4097169734956));
#16793=CARTESIAN_POINT('Ctrl Pts',(-2.51801649770141,0.0601823885902093,
-1.54126937801552));
#16794=CARTESIAN_POINT('Ctrl Pts',(-2.49179296251398,0.592861348991231,
-1.42395434544243));
#16795=CARTESIAN_POINT('Ctrl Pts',(-2.46556942732655,0.956656176813372,
-1.11058164716247));
#16796=CARTESIAN_POINT('Ctrl Pts',(-2.43934589213912,1.32045100463551,-0.797208948882529));
#16797=CARTESIAN_POINT('Ctrl Pts',(-2.41312235695169,1.51536169987877,-0.287778584895738));
#16798=CARTESIAN_POINT('Ctrl Pts',(-2.38689882176426,1.45364820629875,0.188394856012302));
#16799=CARTESIAN_POINT('Ctrl Pts',(-2.36067528657683,1.39193471271873,0.664568296920349));
#16800=CARTESIAN_POINT('Ctrl Pts',(-2.3344517513894,1.07359703031543,1.10748481474964));
#16801=CARTESIAN_POINT('Ctrl Pts',(-2.30822821620197,0.641937119850225,
1.31776417412904));
#16802=CARTESIAN_POINT('Ctrl Pts',(-2.28200468101454,0.21027720938502,1.52804353350844));
#16803=CARTESIAN_POINT('Ctrl Pts',(-2.25578114582711,-0.33470492914208,
1.50568573443795));
#16804=CARTESIAN_POINT('Ctrl Pts',(-2.22955761063968,-0.747697270824022,
1.26076301132885));
#16805=CARTESIAN_POINT('Ctrl Pts',(-2.20333407545225,-1.16068961250596,
1.01584028821975));
#16806=CARTESIAN_POINT('Ctrl Pts',(-2.17711054026482,-1.44169215734274,
0.54835264107206));
#16807=CARTESIAN_POINT('Ctrl Pts',(-2.15088700507739,-1.46419785181459,
0.0687213793496122));
#16808=CARTESIAN_POINT('Ctrl Pts',(-2.14964301866589,-1.46526547209935,
0.0459687349084391));
#16809=CARTESIAN_POINT('Ctrl Pts',(-2.1483990322544,-1.465751385703,0.0231887631643572));
#16810=CARTESIAN_POINT('Ctrl Pts',(-2.14715504584291,-1.46566693596749,
0.000405098676182412));
#16811=CARTESIAN_POINT('Origin',(-8.66086711473615,0.,0.));
#16812=CARTESIAN_POINT('',(-1.91086711473615,-1.17949859053141,0.000362611161451894));
#16813=CARTESIAN_POINT('',(-1.81213288526384,-1.17599517010053,0.000374536726006555));
#16814=CARTESIAN_POINT('',(-8.66086711473615,-1.17775,-9.40918233355216E-14));
#16815=CARTESIAN_POINT('',(-1.6865,1.11895033756726,-0.372858137362636));
#16816=CARTESIAN_POINT('Ctrl Pts',(-1.91086711473615,-1.17949859053141,
0.000362611161451828));
#16817=CARTESIAN_POINT('Ctrl Pts',(-1.88597960410018,-1.17802638490066,
-0.366486395610538));
#16818=CARTESIAN_POINT('Ctrl Pts',(-1.83486855827677,-0.798160605577452,
-1.12254371076134));
#16819=CARTESIAN_POINT('Ctrl Pts',(-1.76007952003139,0.441176614863831,
-1.29467055259558));
#16820=CARTESIAN_POINT('Ctrl Pts',(-1.71017799242198,1.00633421131011,-0.703481264185673));
#16821=CARTESIAN_POINT('Ctrl Pts',(-1.6865,1.11895033756726,-0.372858137362636));
#16822=CARTESIAN_POINT('',(-1.6865,0.00936663037056419,-1.17771275306651));
#16823=CARTESIAN_POINT('Origin',(-1.6865,0.,0.));
#16824=CARTESIAN_POINT('Ctrl Pts',(-1.81213288526384,-1.17599517010053,
0.000374536726006642));
#16825=CARTESIAN_POINT('Ctrl Pts',(-1.79647879202999,-1.17477985141934,
-0.232212701039649));
#16826=CARTESIAN_POINT('Ctrl Pts',(-1.75460116360871,-0.995964068408633,
-0.855730562959772));
#16827=CARTESIAN_POINT('Ctrl Pts',(-1.71272353518743,-0.378730543625381,
-1.1807993824396));
#16828=CARTESIAN_POINT('Ctrl Pts',(-1.6865,0.00936663037056419,-1.17771275306651));
#16829=CARTESIAN_POINT('Origin',(-8.66086711473615,0.,0.));
#16830=CARTESIAN_POINT('',(-2.41086711473615,-1.17697020174115,-0.000948820758233051));
#16831=CARTESIAN_POINT('',(-2.31213288526384,-1.17949383931378,0.000326002709753635));
#16832=CARTESIAN_POINT('',(-8.66086711473615,-1.17775,-9.40918233355216E-14));
#16833=CARTESIAN_POINT('Ctrl Pts',(-2.41086711473615,-1.17697020174115,
-0.000948820758233052));
#16834=CARTESIAN_POINT('Ctrl Pts',(-2.40287768374552,-1.17789239775818,
-0.119358360551166));
#16835=CARTESIAN_POINT('Ctrl Pts',(-2.36866471756746,-1.10738507091887,
-0.625348758528117));
#16836=CARTESIAN_POINT('Ctrl Pts',(-2.30822821620197,-0.384866161144742,
-1.33341914590248));
#16837=CARTESIAN_POINT('Ctrl Pts',(-2.22955761063968,0.902116009207335,
-1.05464830440266));
#16838=CARTESIAN_POINT('Ctrl Pts',(-2.15088700507739,1.37696456000371,0.173588334226353));
#16839=CARTESIAN_POINT('Ctrl Pts',(-2.0722163995151,0.612092873972952,1.24558465502793));
#16840=CARTESIAN_POINT('Ctrl Pts',(-1.9935457939528,-0.703730164986462,
1.19612286163926));
#16841=CARTESIAN_POINT('Ctrl Pts',(-1.93976269902649,-1.1702997645752,0.426214599014237));
#16842=CARTESIAN_POINT('Ctrl Pts',(-1.91220313928761,-1.17957762225525,
0.0200559941957292));
#16843=CARTESIAN_POINT('Ctrl Pts',(-1.91086711473615,-1.17949859053141,
0.000362611161451828));
#16844=CARTESIAN_POINT('Ctrl Pts',(-2.31213288526384,-1.17949383931378,
0.000326002709753667));
#16845=CARTESIAN_POINT('Ctrl Pts',(-2.2871533364879,-1.17812916935092,-0.36784782733973));
#16846=CARTESIAN_POINT('Ctrl Pts',(-2.23595025252454,-0.795963231226945,
-1.12498678959492));
#16847=CARTESIAN_POINT('Ctrl Pts',(-2.15852363337374,0.488222034063068,
-1.29907078650092));
#16848=CARTESIAN_POINT('Ctrl Pts',(-2.07985302781145,1.35367817671458,-0.306589740084279));
#16849=CARTESIAN_POINT('Ctrl Pts',(-2.00118242224916,1.00009581383204,0.962242750523822));
#16850=CARTESIAN_POINT('Ctrl Pts',(-1.92251181668687,-0.253212907927416,
1.36414589400647));
#16851=CARTESIAN_POINT('Ctrl Pts',(-1.85949530435843,-1.07552588043857,
0.703308252629748));
#16852=CARTESIAN_POINT('Ctrl Pts',(-1.82270232721742,-1.17681573760732,
0.157414441368478));
#16853=CARTESIAN_POINT('Ctrl Pts',(-1.81213288526384,-1.17599517010053,
0.000374536726006642));
#16854=CARTESIAN_POINT('Origin',(-8.66086711473615,0.,0.));
#16855=CARTESIAN_POINT('',(-2.91086711473616,-1.17663955749993,0.000844389314044513));
#16856=CARTESIAN_POINT('',(-2.81213288526384,-1.17693457700439,-0.000940564629799273));
#16857=CARTESIAN_POINT('',(-8.66086711473615,-1.17775,-9.40918233355216E-14));
#16858=CARTESIAN_POINT('Ctrl Pts',(-2.91086711473616,-1.17663955749993,
0.000844389314044337));
#16859=CARTESIAN_POINT('Ctrl Pts',(-2.89355222820344,-1.17489737407618,
-0.255957831126769));
#16860=CARTESIAN_POINT('Ctrl Pts',(-2.85001380648329,-0.966594683781144,
-0.904261982661384));
#16861=CARTESIAN_POINT('Ctrl Pts',(-2.78025184957571,0.0978503055697247,
-1.38439494624008));
#16862=CARTESIAN_POINT('Ctrl Pts',(-2.70158124401342,1.21013193153834,-0.679488016032942));
#16863=CARTESIAN_POINT('Ctrl Pts',(-2.62291063845113,1.232947968949,0.637152805391334));
#16864=CARTESIAN_POINT('Ctrl Pts',(-2.54424003288884,0.145755609165987,
1.38017397139449));
#16865=CARTESIAN_POINT('Ctrl Pts',(-2.47355885831718,-0.948919964424747,
0.931371035446015));
#16866=CARTESIAN_POINT('Ctrl Pts',(-2.42910121893295,-1.17486549387346,
0.269294690827376));
#16867=CARTESIAN_POINT('Ctrl Pts',(-2.41086711473615,-1.17697020174115,
-0.000948820758233052));
#16868=CARTESIAN_POINT('Ctrl Pts',(-2.81213288526384,-1.17693457700439,
-0.000940564629799308));
#16869=CARTESIAN_POINT('Ctrl Pts',(-2.80405141613325,-1.17785678127362,
-0.120723243775803));
#16870=CARTESIAN_POINT('Ctrl Pts',(-2.76974641181523,-1.10631193161732,
-0.62811326056394));
#16871=CARTESIAN_POINT('Ctrl Pts',(-2.70921787230977,-0.38024109152726,
-1.33474396280885));
#16872=CARTESIAN_POINT('Ctrl Pts',(-2.63054726674748,0.905777314237609,
-1.05151653620214));
#16873=CARTESIAN_POINT('Ctrl Pts',(-2.5518766611852,1.37633981097026,0.178374023112081));
#16874=CARTESIAN_POINT('Ctrl Pts',(-2.4732060556229,0.607794121628612,1.24768375090184));
#16875=CARTESIAN_POINT('Ctrl Pts',(-2.39453545006062,-0.707927190944584,
1.19370650897096));
#16876=CARTESIAN_POINT('Ctrl Pts',(-2.34084439327426,-1.17092757672768,
0.423439602299549));
#16877=CARTESIAN_POINT('Ctrl Pts',(-2.31337687167533,-1.17956180014466,
0.018661131408755));
#16878=CARTESIAN_POINT('Ctrl Pts',(-2.31213288526384,-1.17949383931378,
0.000326002709753667));
#16879=CARTESIAN_POINT('Origin',(-8.66086711473615,0.,0.));
#16880=CARTESIAN_POINT('',(-3.41086711473615,-1.17959136717079,-0.000110183320623983));
#16881=CARTESIAN_POINT('',(-3.31213288526384,-1.17667046800503,0.000856680601965393));
#16882=CARTESIAN_POINT('',(-8.66086711473615,-1.17775,-9.40918233355216E-14));
#16883=CARTESIAN_POINT('Ctrl Pts',(-3.41086711473615,-1.17959136717079,
-0.000110183320623943));
#16884=CARTESIAN_POINT('Ctrl Pts',(-3.41045030784878,-1.17959970513283,
-0.00625203394745172));
#16885=CARTESIAN_POINT('Ctrl Pts',(-3.38380996577397,-1.1767938832024,-0.398802509579523));
#16886=CARTESIAN_POINT('Ctrl Pts',(-3.33094608851175,-0.744809034162001,
-1.17106078215508));
#16887=CARTESIAN_POINT('Ctrl Pts',(-3.25227548294945,0.568601241925253,
-1.26602388853876));
#16888=CARTESIAN_POINT('Ctrl Pts',(-3.17360487738716,1.37010712465924,-0.22120196322891));
#16889=CARTESIAN_POINT('Ctrl Pts',(-3.09493427182487,0.938123194652226,
1.02276523601594));
#16890=CARTESIAN_POINT('Ctrl Pts',(-3.01626366626258,-0.338441009250009,
1.34595006244152));
#16891=CARTESIAN_POINT('Ctrl Pts',(-2.95490794723301,-1.09640882153771,
0.652958858257086));
#16892=CARTESIAN_POINT('Ctrl Pts',(-2.91977576339087,-1.17753592491099,
0.132971201195474));
#16893=CARTESIAN_POINT('Ctrl Pts',(-2.91086711473616,-1.17663955749993,
0.000844389314044337));
#16894=CARTESIAN_POINT('Ctrl Pts',(-3.31213288526384,-1.17667046800503,
0.000856680601965358));
#16895=CARTESIAN_POINT('Ctrl Pts',(-3.29472596059116,-1.17489029018727,
-0.257293424885117));
#16896=CARTESIAN_POINT('Ctrl Pts',(-3.25109550073105,-0.964857764256308,
-0.906981790783454));
#16897=CARTESIAN_POINT('Ctrl Pts',(-3.18124150568352,0.102653133571944,
-1.38404698750922));
#16898=CARTESIAN_POINT('Ctrl Pts',(-3.10257090012123,1.2124824062959,-0.675285143647363));
#16899=CARTESIAN_POINT('Ctrl Pts',(-3.02390029455893,1.23072943933634,0.641427153820911));
#16900=CARTESIAN_POINT('Ctrl Pts',(-2.94522968899665,0.140966433426828,
1.38067098062933));
#16901=CARTESIAN_POINT('Ctrl Pts',(-2.87464055256494,-0.950723338242491,
0.928662811933087));
#16902=CARTESIAN_POINT('Ctrl Pts',(-2.83027495132068,-1.17486432337848,
0.267959216142224));
#16903=CARTESIAN_POINT('Ctrl Pts',(-2.81213288526384,-1.17693457700439,
-0.000940564629799308));
#16904=CARTESIAN_POINT('Origin',(-8.66086711473615,0.,0.));
#16905=CARTESIAN_POINT('',(-3.91086711473616,-1.17638334390667,-0.000716697455210677));
#16906=CARTESIAN_POINT('',(-3.81213288526384,-1.17958479253191,-0.000134358022525483));
#16907=CARTESIAN_POINT('',(-8.66086711473615,-1.17775,-9.40918233355216E-14));
#16908=CARTESIAN_POINT('Ctrl Pts',(-3.91086711473616,-1.17638334390667,
-0.000716697455210805));
#16909=CARTESIAN_POINT('Ctrl Pts',(-3.9011248523067,-1.17720337900645,-0.145286422711667));
#16910=CARTESIAN_POINT('Ctrl Pts',(-3.86515905468981,-1.08593957103214,
-0.677999935594477));
#16911=CARTESIAN_POINT('Ctrl Pts',(-3.80296972188548,-0.295982347342492,
-1.35591972587991));
#16912=CARTESIAN_POINT('Ctrl Pts',(-3.72429911632319,0.969796609117977,
-0.992783153602477));
#16913=CARTESIAN_POINT('Ctrl Pts',(-3.6456285107609,1.36248014896398,0.264143325656574));
#16914=CARTESIAN_POINT('Ctrl Pts',(-3.56695790519861,0.528540331258045,
1.28326496528333));
#16915=CARTESIAN_POINT('Ctrl Pts',(-3.4887041065237,-0.774298180626516,
1.14780118577342));
#16916=CARTESIAN_POINT('Ctrl Pts',(-3.43667384303621,-1.17907511965292,
0.380164411911229));
#16917=CARTESIAN_POINT('Ctrl Pts',(-3.41086711473615,-1.17959136717079,
-0.000110183320623943));
#16918=CARTESIAN_POINT('Ctrl Pts',(-3.81213288526384,-1.17958479253191,
-0.000134358022525584));
#16919=CARTESIAN_POINT('Ctrl Pts',(-3.8116240402365,-1.17959709699341,-0.00763254663005804));
#16920=CARTESIAN_POINT('Ctrl Pts',(-3.78489166002174,-1.17615977017934,
-0.401541357004618));
#16921=CARTESIAN_POINT('Ctrl Pts',(-3.73193574461955,-0.740741232249389,
-1.17363798581818));
#16922=CARTESIAN_POINT('Ctrl Pts',(-3.65326513905726,0.572990579286003,
-1.26404331095425));
#16923=CARTESIAN_POINT('Ctrl Pts',(-3.57459453349497,1.3708663395606,-0.216446696849244));
#16924=CARTESIAN_POINT('Ctrl Pts',(-3.49592392793268,0.934568764120381,
1.02601409348018));
#16925=CARTESIAN_POINT('Ctrl Pts',(-3.41725332237039,-0.34310905511451,
1.34476759219195));
#16926=CARTESIAN_POINT('Ctrl Pts',(-3.35598964148077,-1.09753440075601,
0.65019412424173));
#16927=CARTESIAN_POINT('Ctrl Pts',(-3.32094949577859,-1.17757212839372,
0.131609756014222));
#16928=CARTESIAN_POINT('Ctrl Pts',(-3.31213288526384,-1.17667046800503,
0.000856680601965358));
#16929=CARTESIAN_POINT('Origin',(-8.66086711473615,0.,0.));
#16930=CARTESIAN_POINT('',(-4.41086711473616,-1.17730203530188,0.00100741500783658));
#16931=CARTESIAN_POINT('',(-4.31213288526384,-1.17635786578603,-0.000700921021541262));
#16932=CARTESIAN_POINT('',(-8.66086711473615,-1.17775,-9.40918233355216E-14));
#16933=CARTESIAN_POINT('Ctrl Pts',(-4.41086711473616,-1.17730203530188,
0.00100741500783666));
#16934=CARTESIAN_POINT('Ctrl Pts',(-4.39179939676461,-1.17491412509447,
-0.28138822708182));
#16935=CARTESIAN_POINT('Ctrl Pts',(-4.34650814360563,-0.932258082234428,
-0.955843334036929));
#16936=CARTESIAN_POINT('Ctrl Pts',(-4.27499335525923,0.189051166264626,
-1.37491218247906));
#16937=CARTESIAN_POINT('Ctrl Pts',(-4.19632274969693,1.25235902888845,-0.598097580467343));
#16938=CARTESIAN_POINT('Ctrl Pts',(-4.11765214413465,1.18818416202297,0.717176582238888));
#16939=CARTESIAN_POINT('Ctrl Pts',(-4.03898153857235,0.0543023730844936,
1.38678589020371));
#16940=CARTESIAN_POINT('Ctrl Pts',(-3.97005319543952,-0.981997558039448,
0.879577951977616));
#16941=CARTESIAN_POINT('Ctrl Pts',(-3.92734838749413,-1.17499606633655,
0.243856171706187));
#16942=CARTESIAN_POINT('Ctrl Pts',(-3.91086711473616,-1.17638334390667,
-0.000716697455210805));
#16943=CARTESIAN_POINT('Ctrl Pts',(-4.31213288526384,-1.17635786578603,
-0.000700921021541401));
#16944=CARTESIAN_POINT('Ctrl Pts',(-4.30229858469442,-1.17716630005596,
-0.146644373245256));
#16945=CARTESIAN_POINT('Ctrl Pts',(-4.26624074893757,-1.08475308443882,
-0.680764528174929));
#16946=CARTESIAN_POINT('Ctrl Pts',(-4.20395937799329,-0.29127585234018,
-1.35693849265711));
#16947=CARTESIAN_POINT('Ctrl Pts',(-4.125288772431,0.973235439907126,-0.989412185868934));
#16948=CARTESIAN_POINT('Ctrl Pts',(-4.04661816686871,1.36155538052876,0.268869188915402));
#16949=CARTESIAN_POINT('Ctrl Pts',(-3.96794756130642,0.524084520485498,
1.28509109030307));
#16950=CARTESIAN_POINT('Ctrl Pts',(-3.88978580077146,-0.776744299388545,
1.14527225033765));
#16951=CARTESIAN_POINT('Ctrl Pts',(-3.83784757542394,-1.1789629815715,0.378789649184804));
#16952=CARTESIAN_POINT('Ctrl Pts',(-3.81213288526384,-1.17958479253191,
-0.000134358022525584));
#16953=CARTESIAN_POINT('Origin',(-8.66086711473615,0.,0.));
#16954=CARTESIAN_POINT('',(-4.91086711473616,-1.17927992659326,-0.000541138395992998));
#16955=CARTESIAN_POINT('',(-4.81213288526384,-1.1773401869437,0.00101152320117252));
#16956=CARTESIAN_POINT('',(-8.66086711473615,-1.17775,-9.40918233355216E-14));
#16957=CARTESIAN_POINT('Ctrl Pts',(-4.91086711473616,-1.17927992659326,
-0.000541138395993047));
#16958=CARTESIAN_POINT('Ctrl Pts',(-4.90869747640996,-1.1794645160417,-0.0325343443996988));
#16959=CARTESIAN_POINT('Ctrl Pts',(-4.88030430289632,-1.16387484001231,
-0.451033884711238));
#16960=CARTESIAN_POINT('Ctrl Pts',(-4.82568759419526,-0.66585587424462,
-1.21768625176223));
#16961=CARTESIAN_POINT('Ctrl Pts',(-4.74701698863296,0.650958493169218,
-1.22571484985989));
#16962=CARTESIAN_POINT('Ctrl Pts',(-4.66834638307068,1.38172329992943,-0.130248130230639));
#16963=CARTESIAN_POINT('Ctrl Pts',(-4.58967577750838,0.868540387494536,
1.08247930617046));
#16964=CARTESIAN_POINT('Ctrl Pts',(-4.5110051719461,-0.42657826714551,1.32066454294621));
#16965=CARTESIAN_POINT('Ctrl Pts',(-4.45140228435535,-1.1168328254269,0.60031985529612));
#16966=CARTESIAN_POINT('Ctrl Pts',(-4.41802293195204,-1.17819818076604,
0.106986095853185));
#16967=CARTESIAN_POINT('Ctrl Pts',(-4.41086711473616,-1.17730203530188,
0.00100741500783666));
#16968=CARTESIAN_POINT('Ctrl Pts',(-4.81213288526384,-1.1773401869437,0.00101152320117258));
#16969=CARTESIAN_POINT('Ctrl Pts',(-4.79297312915233,-1.17492446024765,
-0.282723747894919));
#16970=CARTESIAN_POINT('Ctrl Pts',(-4.7475898378534,-0.930380861478271,
-0.958537919647446));
#16971=CARTESIAN_POINT('Ctrl Pts',(-4.67598301136704,0.193820620708426,
-1.37424788957624));
#16972=CARTESIAN_POINT('Ctrl Pts',(-4.59731240580474,1.25442668732974,-0.593748584109574));
#16973=CARTESIAN_POINT('Ctrl Pts',(-4.51864180024246,1.18568853815801,0.721294936553209));
#16974=CARTESIAN_POINT('Ctrl Pts',(-4.43997119468016,0.049490244982279,
1.38696590104707));
#16975=CARTESIAN_POINT('Ctrl Pts',(-4.37113488968729,-0.983662136505136,
0.876847394213616));
#16976=CARTESIAN_POINT('Ctrl Pts',(-4.32852211988185,-1.1750105794356,0.242519373352494));
#16977=CARTESIAN_POINT('Ctrl Pts',(-4.31213288526384,-1.17635786578603,
-0.000700921021541401));
#16978=CARTESIAN_POINT('Origin',(-8.66086711473615,0.,0.));
#16979=CARTESIAN_POINT('',(-5.41086711473616,-1.17600992997557,-0.000371065616479655));
#16980=CARTESIAN_POINT('',(-5.31213288526384,-1.17925411379821,-0.000561242925713745));
#16981=CARTESIAN_POINT('',(-8.66086711473615,-1.17775,-9.40918233355216E-14));
#16982=CARTESIAN_POINT('Ctrl Pts',(-5.41086711473616,-1.17600992997557,
-0.000371065616479732));
#16983=CARTESIAN_POINT('Ctrl Pts',(-5.39937202086787,-1.17650112810648,
-0.171087869735001));
#16984=CARTESIAN_POINT('Ctrl Pts',(-5.36165339181215,-1.06227811533873,
-0.730631560415982));
#16985=CARTESIAN_POINT('Ctrl Pts',(-5.297711227569,-0.205802127560476,-1.37250476768144));
#16986=CARTESIAN_POINT('Ctrl Pts',(-5.21904062200671,1.03323559121881,-0.926578688525379));
#16987=CARTESIAN_POINT('Ctrl Pts',(-5.14037001644442,1.34206459371129,0.353534268919763));
#16988=CARTESIAN_POINT('Ctrl Pts',(-5.06169941088212,0.442650100242435,
1.31536487019939));
#16989=CARTESIAN_POINT('Ctrl Pts',(-4.98519844364604,-0.819481368292237,
1.09912223479354));
#16990=CARTESIAN_POINT('Ctrl Pts',(-4.93492101159739,-1.17723345852483,
0.354154512109054));
#16991=CARTESIAN_POINT('Ctrl Pts',(-4.91086711473616,-1.17927992659326,
-0.000541138395993047));
#16992=CARTESIAN_POINT('Ctrl Pts',(-5.31213288526384,-1.17925411379821,
-0.000561242925713546));
#16993=CARTESIAN_POINT('Ctrl Pts',(-5.30987120879768,-1.17945240900491,
-0.0339135600639547));
#16994=CARTESIAN_POINT('Ctrl Pts',(-5.28138599714409,-1.16314653333968,
-0.45378048918944));
#16995=CARTESIAN_POINT('Ctrl Pts',(-5.22667725030306,-0.66162677306598,
-1.21998922461717));
#16996=CARTESIAN_POINT('Ctrl Pts',(-5.14800664474078,0.655207470874117,
-1.22344875868442));
#16997=CARTESIAN_POINT('Ctrl Pts',(-5.06933603917847,1.38216685417029,-0.12545310777169));
#16998=CARTESIAN_POINT('Ctrl Pts',(-4.9906654336162,0.86477919209241,1.08548636285362));
#16999=CARTESIAN_POINT('Ctrl Pts',(-4.9119948280539,-0.431158056335988,
1.31917641938943));
#17000=CARTESIAN_POINT('Ctrl Pts',(-4.85248397860312,-1.11784699831804,
0.597557127533712));
#17001=CARTESIAN_POINT('Ctrl Pts',(-4.81919666433976,-1.17823081204297,
0.105618453446316));
#17002=CARTESIAN_POINT('Ctrl Pts',(-4.81213288526384,-1.1773401869437,0.00101152320117258));
#17003=CARTESIAN_POINT('Origin',(-8.66086711473615,0.,0.));
#17004=CARTESIAN_POINT('',(-5.91086711473616,-1.1780553849581,0.00100231958302903));
#17005=CARTESIAN_POINT('',(-5.81213288526384,-1.17599715609266,-0.000350803616455952));
#17006=CARTESIAN_POINT('',(-8.66086711473615,-1.17775,-9.40918233355216E-14));
#17007=CARTESIAN_POINT('Ctrl Pts',(-5.91086711473616,-1.1780553849581,0.00100231958302903));
#17008=CARTESIAN_POINT('Ctrl Pts',(-5.89004656532578,-1.17529941481109,
-0.306848134423301));
#17009=CARTESIAN_POINT('Ctrl Pts',(-5.84300248072798,-0.895208689127834,
-1.0068819708241));
#17010=CARTESIAN_POINT('Ctrl Pts',(-5.76973486094274,0.279426911638065,
-1.3594279881432));
#17011=CARTESIAN_POINT('Ctrl Pts',(-5.69106425538045,1.28911939778457,-0.514096324773416));
#17012=CARTESIAN_POINT('Ctrl Pts',(-5.61239364981816,1.13823426692583,0.794069648334226));
#17013=CARTESIAN_POINT('Ctrl Pts',(-5.53372304425587,-0.0373885377105224,
1.38734492840875));
#17014=CARTESIAN_POINT('Ctrl Pts',(-5.46654753256187,-1.01249108072428,
0.827425065489171));
#17015=CARTESIAN_POINT('Ctrl Pts',(-5.4255955560553,-1.17538056731615,0.218365071770556));
#17016=CARTESIAN_POINT('Ctrl Pts',(-5.41086711473616,-1.17600992997557,
-0.000371065616479732));
#17017=CARTESIAN_POINT('Ctrl Pts',(-5.81213288526384,-1.17599715609266,
-0.000350803616455952));
#17018=CARTESIAN_POINT('Ctrl Pts',(-5.80054575325559,-1.17646494966617,
-0.172439149737962));
#17019=CARTESIAN_POINT('Ctrl Pts',(-5.76273508605991,-1.06097257609266,
-0.733393343710012));
#17020=CARTESIAN_POINT('Ctrl Pts',(-5.69870088367681,-0.201038633207167,
-1.37321053124158));
#17021=CARTESIAN_POINT('Ctrl Pts',(-5.62003027811452,1.03644432469548,-0.922988004686612));
#17022=CARTESIAN_POINT('Ctrl Pts',(-5.54135967255223,1.34082978479473,0.358188753595292));
#17023=CARTESIAN_POINT('Ctrl Pts',(-5.46268906698994,0.438083431536926,
1.31689278305031));
#17024=CARTESIAN_POINT('Ctrl Pts',(-5.3862801378938,-0.821772524436675,
1.09653760690973));
#17025=CARTESIAN_POINT('Ctrl Pts',(-5.33609474398511,-1.17715322899035,
0.352797658424898));
#17026=CARTESIAN_POINT('Ctrl Pts',(-5.31213288526384,-1.17925411379821,
-0.000561242925713546));
#17027=CARTESIAN_POINT('Origin',(-8.66086711473615,0.,0.));
#17028=CARTESIAN_POINT('',(-6.41086711473616,-1.17867790410982,-0.000859279010538999));
#17029=CARTESIAN_POINT('',(-6.31213288526384,-1.17809532958918,0.000997103128024986));
#17030=CARTESIAN_POINT('',(-8.66086711473615,-1.17775,-9.40918233355216E-14));
#17031=CARTESIAN_POINT('Ctrl Pts',(-6.41086711473616,-1.17867790410982,
-0.000859279010538855));
#17032=CARTESIAN_POINT('Ctrl Pts',(-6.40694464497113,-1.17915438960473,
-0.0587771547817094));
#17033=CARTESIAN_POINT('Ctrl Pts',(-6.37679864001867,-1.14912484901267,
-0.503407322287921));
#17034=CARTESIAN_POINT('Ctrl Pts',(-6.32042909987877,-0.583996247497372,
-1.25899648606665));
#17035=CARTESIAN_POINT('Ctrl Pts',(-6.24175849431649,0.73047430811023,-1.18005558026704));
#17036=CARTESIAN_POINT('Ctrl Pts',(-6.1630878887542,1.38730824708363,-0.0387257526847742));
#17037=CARTESIAN_POINT('Ctrl Pts',(-6.0844172831919,0.795166405654621,1.1374683419316));
#17038=CARTESIAN_POINT('Ctrl Pts',(-6.00574667762961,-0.512853522972119,
1.28961433097063));
#17039=CARTESIAN_POINT('Ctrl Pts',(-5.9478966214777,-1.13517951613434,0.547741260286263));
#17040=CARTESIAN_POINT('Ctrl Pts',(-5.91627010051321,-1.17877056625389,
0.0808902990821281));
#17041=CARTESIAN_POINT('Ctrl Pts',(-5.91086711473616,-1.1780553849581,0.00100231958302903));
#17042=CARTESIAN_POINT('Ctrl Pts',(-6.31213288526384,-1.17809532958918,
0.000997103128024977));
#17043=CARTESIAN_POINT('Ctrl Pts',(-6.2912202977135,-1.17533124755718,-0.308187145896592));
#17044=CARTESIAN_POINT('Ctrl Pts',(-6.24408417497574,-0.89318672921757,
-1.00954427203146));
#17045=CARTESIAN_POINT('Ctrl Pts',(-6.17072451705056,0.284142091338451,
-1.35845020984985));
#17046=CARTESIAN_POINT('Ctrl Pts',(-6.09205391148824,1.29089537055166,-0.509620287250948));
#17047=CARTESIAN_POINT('Ctrl Pts',(-6.01338330592598,1.13547214593956,0.798014222500227));
#17048=CARTESIAN_POINT('Ctrl Pts',(-5.93471270036367,-0.0422020497217742,
1.38720679169256));
#17049=CARTESIAN_POINT('Ctrl Pts',(-5.86762922680964,-1.01402256959767,
0.824678746007463));
#17050=CARTESIAN_POINT('Ctrl Pts',(-5.82676928844302,-1.17540625790132,
0.217024334120822));
#17051=CARTESIAN_POINT('Ctrl Pts',(-5.81213288526384,-1.17599715609266,
-0.000350803616455952));
#17052=CARTESIAN_POINT('Origin',(-8.66086711473615,0.,0.));
#17053=CARTESIAN_POINT('',(-6.91086711473616,-1.17589437083333,3.29986289264394E-5));
#17054=CARTESIAN_POINT('',(-6.81213288526384,-1.17864116107843,-0.000871798980908167));
#17055=CARTESIAN_POINT('',(-8.66086711473615,-1.17775,-9.40918233355216E-14));
#17056=CARTESIAN_POINT('Ctrl Pts',(-6.91086711473616,-1.17589467053987,
3.29932992490858E-5));
#17057=CARTESIAN_POINT('Ctrl Pts',(-6.89761918942904,-1.17584631531485,
-0.196764413629324));
#17058=CARTESIAN_POINT('Ctrl Pts',(-6.8581477289345,-1.03630390526793,-0.783176720222471));
#17059=CARTESIAN_POINT('Ctrl Pts',(-6.79245273325251,-0.114723332390545,
-1.38309735453967));
#17060=CARTESIAN_POINT('Ctrl Pts',(-6.71378212769023,1.09216436667117,-0.856330476563782));
#17061=CARTESIAN_POINT('Ctrl Pts',(-6.63511152212794,1.31579099157645,0.441382439659493));
#17062=CARTESIAN_POINT('Ctrl Pts',(-6.55644091656565,0.354827664455788,
1.34172299085838));
#17063=CARTESIAN_POINT('Ctrl Pts',(-6.48169278076838,-0.861741836051922,
1.04946482550319));
#17064=CARTESIAN_POINT('Ctrl Pts',(-6.43316818015856,-1.1759688624011,0.32843078925572));
#17065=CARTESIAN_POINT('Ctrl Pts',(-6.41086711473616,-1.17867790410982,
-0.000859279010538855));
#17066=CARTESIAN_POINT('Ctrl Pts',(-6.81213288526384,-1.17864116107843,
-0.000871798980908263));
#17067=CARTESIAN_POINT('Ctrl Pts',(-6.80811837735885,-1.17913357190592,
-0.0601535095849911));
#17068=CARTESIAN_POINT('Ctrl Pts',(-6.77788033426643,-1.14829825666904,
-0.506161144387834));
#17069=CARTESIAN_POINT('Ctrl Pts',(-6.72141875598658,-0.579624239257938,
-1.26101500289363));
#17070=CARTESIAN_POINT('Ctrl Pts',(-6.64274815042429,0.734564342461029,
-1.17751395698303));
#17071=CARTESIAN_POINT('Ctrl Pts',(-6.564077544862,1.38743422631486,-0.0339118586638691));
#17072=CARTESIAN_POINT('Ctrl Pts',(-6.4854069392997,0.791214847056285,1.14022045088028));
#17073=CARTESIAN_POINT('Ctrl Pts',(-6.40673633373742,-0.517325047723218,
1.28782705533921));
#17074=CARTESIAN_POINT('Ctrl Pts',(-6.34897831572546,-1.1360871562569,0.544982882691587));
#17075=CARTESIAN_POINT('Ctrl Pts',(-6.31744383290093,-1.17879729413093,
0.0795173413736451));
#17076=CARTESIAN_POINT('Ctrl Pts',(-6.31213288526384,-1.17809532958918,
0.000997103128024977));
#17077=CARTESIAN_POINT('Origin',(-8.66086711473615,0.,0.));
#17078=CARTESIAN_POINT('',(-7.41086711473616,-1.17877062515776,0.000899836917228718));
#17079=CARTESIAN_POINT('',(-7.31213288526384,-1.17589382943587,6.0515499218719E-5));
#17080=CARTESIAN_POINT('',(-8.66086711473615,-1.17775,-9.40918233355216E-14));
#17081=CARTESIAN_POINT('Ctrl Pts',(-7.41086711473616,-1.17877062515776,
0.00089983691722877));
#17082=CARTESIAN_POINT('Ctrl Pts',(-7.38829373388695,-1.17611490904963,
-0.33232246422372));
#17083=CARTESIAN_POINT('Ctrl Pts',(-7.33949681785032,-0.855386430900654,
-1.05736004564147));
#17084=CARTESIAN_POINT('Ctrl Pts',(-7.26447636662626,0.368594759353147,
-1.33794018873242));
#17085=CARTESIAN_POINT('Ctrl Pts',(-7.18580576106397,1.32024655518524,-0.427887663681729));
#17086=CARTESIAN_POINT('Ctrl Pts',(-7.10713515550168,1.0833192355362,0.867515846081762));
#17087=CARTESIAN_POINT('Ctrl Pts',(-7.02846454993939,-0.128917960242522,
1.38183808732227));
#17088=CARTESIAN_POINT('Ctrl Pts',(-6.96304186968421,-1.04049409675069,
0.775023379664861));
#17089=CARTESIAN_POINT('Ctrl Pts',(-6.92384272461647,-1.17594203180746,
0.192785165323541));
#17090=CARTESIAN_POINT('Ctrl Pts',(-6.91086711473616,-1.17589467053987,
3.29932992490858E-5));
#17091=CARTESIAN_POINT('Ctrl Pts',(-7.31213288526384,-1.17589382943587,
6.05154992187017E-5));
#17092=CARTESIAN_POINT('Ctrl Pts',(-7.29879292181676,-1.17581348019214,
-0.198106859471453));
#17093=CARTESIAN_POINT('Ctrl Pts',(-7.25922942318226,-1.03487877075373,
-0.785943419169282));
#17094=CARTESIAN_POINT('Ctrl Pts',(-7.19344238936034,-0.109920457047265,
-1.38347881456886));
#17095=CARTESIAN_POINT('Ctrl Pts',(-7.11477178379802,1.095127328248,-0.852540070304724));
#17096=CARTESIAN_POINT('Ctrl Pts',(-7.03610117823576,1.31425240912282,0.445947499710114));
#17097=CARTESIAN_POINT('Ctrl Pts',(-6.95743057267344,0.350169610287078,
1.34294482869753));
#17098=CARTESIAN_POINT('Ctrl Pts',(-6.88277447501615,-0.863881069525856,
1.04683402745875));
#17099=CARTESIAN_POINT('Ctrl Pts',(-6.83434191254628,-1.17591704998917,
0.327085987954644));
#17100=CARTESIAN_POINT('Ctrl Pts',(-6.81213288526384,-1.17864116107843,
-0.000871798980908263));
#17101=CARTESIAN_POINT('Origin',(-1.6865,3.28582941601228E-17,0.));
#17102=CARTESIAN_POINT('',(-1.6865,-0.26238990830909,1.43978602091337));
#17103=CARTESIAN_POINT('Ctrl Pts',(-1.6865,1.11895033756726,-0.372858137362636));
#17104=CARTESIAN_POINT('Ctrl Pts',(-1.6865,1.13535536132518,-0.338481041248113));
#17105=CARTESIAN_POINT('Ctrl Pts',(-1.6865,1.14996080409863,-0.303357275824646));
#17106=CARTESIAN_POINT('Ctrl Pts',(-1.6865,1.16267058779846,-0.267595343165902));
#17107=CARTESIAN_POINT('Ctrl Pts',(-1.6865,1.17888071541452,-0.221984378739937));
#17108=CARTESIAN_POINT('Ctrl Pts',(-1.6865,1.19200950533875,-0.175335963428926));
#17109=CARTESIAN_POINT('Ctrl Pts',(-1.6865,1.20217294148064,-0.127929909118842));
#17110=CARTESIAN_POINT('Ctrl Pts',(-1.6865,1.20592469774747,-0.110430319525292));
#17111=CARTESIAN_POINT('Ctrl Pts',(-1.6865,1.2092719382956,-0.0928272229185943));
#17112=CARTESIAN_POINT('Ctrl Pts',(-1.6865,1.21221895595122,-0.0751338976379057));
#17113=CARTESIAN_POINT('Ctrl Pts',(-1.6865,1.21398506969953,-0.0645304915225663));
#17114=CARTESIAN_POINT('Ctrl Pts',(-1.6865,1.21560669230278,-0.0538986526621468));
#17115=CARTESIAN_POINT('Ctrl Pts',(-1.6865,1.21708402895976,-0.0432493233469738));
#17116=CARTESIAN_POINT('Ctrl Pts',(-1.6865,1.22403289104792,0.00684130453578788));
#17117=CARTESIAN_POINT('Ctrl Pts',(-1.6865,1.22780217473515,0.0573687104521416));
#17118=CARTESIAN_POINT('Ctrl Pts',(-1.6865,1.22852178751262,0.108025567468149));
#17119=CARTESIAN_POINT('Ctrl Pts',(-1.6865,1.2290363948802,0.144251149690937));
#17120=CARTESIAN_POINT('Ctrl Pts',(-1.6865,1.22799041925717,0.180543667430809));
#17121=CARTESIAN_POINT('Ctrl Pts',(-1.6865,1.22541633213672,0.216796772140719));
#17122=CARTESIAN_POINT('Ctrl Pts',(-1.6865,1.22459563153091,0.228355411613986));
#17123=CARTESIAN_POINT('Ctrl Pts',(-1.6865,1.22361949764788,0.239910068294751));
#17124=CARTESIAN_POINT('Ctrl Pts',(-1.6865,1.22248871598296,0.251457345648952));
#17125=CARTESIAN_POINT('Ctrl Pts',(-1.6865,1.22157697590322,0.26076782166951));
#17126=CARTESIAN_POINT('Ctrl Pts',(-1.6865,1.22056477417449,0.270071996499609));
#17127=CARTESIAN_POINT('Ctrl Pts',(-1.6865,1.21945390680089,0.279358560962091));
#17128=CARTESIAN_POINT('Ctrl Pts',(-1.6865,1.21322430593567,0.331436415965335));
#17129=CARTESIAN_POINT('Ctrl Pts',(-1.6865,1.20388812344957,0.383041243620923));
#17130=CARTESIAN_POINT('Ctrl Pts',(-1.6865,1.1915757568237,0.433859467629619));
#17131=CARTESIAN_POINT('Ctrl Pts',(-1.6865,1.17901846548233,0.485688597131582));
#17132=CARTESIAN_POINT('Ctrl Pts',(-1.6865,1.16336550530721,0.536700681103785));
#17133=CARTESIAN_POINT('Ctrl Pts',(-1.6865,1.14470297529775,0.586573510429021));
#17134=CARTESIAN_POINT('Ctrl Pts',(-1.6865,1.13355797389477,0.616356865232393));
#17135=CARTESIAN_POINT('Ctrl Pts',(-1.6865,1.12133866272013,0.645734045864069));
#17136=CARTESIAN_POINT('Ctrl Pts',(-1.6865,1.10805456343179,0.674635440120251));
#17137=CARTESIAN_POINT('Ctrl Pts',(-1.6865,1.10137874179942,0.689159612876959));
#17138=CARTESIAN_POINT('Ctrl Pts',(-1.6865,1.09443390630556,0.703563601099449));
#17139=CARTESIAN_POINT('Ctrl Pts',(-1.6865,1.08722064460436,0.717838352010837));
#17140=CARTESIAN_POINT('Ctrl Pts',(-1.6865,1.08181939494862,0.728527204937547));
#17141=CARTESIAN_POINT('Ctrl Pts',(-1.6865,1.07626632906913,0.739145673762293));
#17142=CARTESIAN_POINT('Ctrl Pts',(-1.6865,1.07057335460936,0.749669029712744));
#17143=CARTESIAN_POINT('Ctrl Pts',(-1.6865,1.04448849650432,0.797886398101832));
#17144=CARTESIAN_POINT('Ctrl Pts',(-1.6865,1.01542414332133,0.844202514930974));
#17145=CARTESIAN_POINT('Ctrl Pts',(-1.6865,0.98348603073344,0.888285135110482));
#17146=CARTESIAN_POINT('Ctrl Pts',(-1.6865,0.976132732681375,0.898434534020762));
#17147=CARTESIAN_POINT('Ctrl Pts',(-1.6865,0.968626883363404,0.908465522082479));
#17148=CARTESIAN_POINT('Ctrl Pts',(-1.6865,0.960969385665994,0.918373986113659));
#17149=CARTESIAN_POINT('Ctrl Pts',(-1.6865,0.928822249709468,0.959970961120058));
#17150=CARTESIAN_POINT('Ctrl Pts',(-1.6865,0.894006124211354,0.999410536617324));
#17151=CARTESIAN_POINT('Ctrl Pts',(-1.6865,0.856811235932228,1.03663507024378));
#17152=CARTESIAN_POINT('Ctrl Pts',(-1.6865,0.838875125773088,1.05458547597524));
#17153=CARTESIAN_POINT('Ctrl Pts',(-1.6865,0.820385172914883,1.07202043593171));
#17154=CARTESIAN_POINT('Ctrl Pts',(-1.6865,0.801370429731241,1.08893116790782));
#17155=CARTESIAN_POINT('Ctrl Pts',(-1.6865,0.789265686005685,1.09969650272226));
#17156=CARTESIAN_POINT('Ctrl Pts',(-1.6865,0.776948224556874,1.1102493585158));
#17157=CARTESIAN_POINT('Ctrl Pts',(-1.6865,0.764425135746565,1.12058710188661));
#17158=CARTESIAN_POINT('Ctrl Pts',(-1.6865,0.756948856335036,1.12675873087492));
#17159=CARTESIAN_POINT('Ctrl Pts',(-1.6865,0.749400063604347,1.13285292413839));
#17160=CARTESIAN_POINT('Ctrl Pts',(-1.6865,0.741790382865105,1.13886148265789));
#17161=CARTESIAN_POINT('Ctrl Pts',(-1.6865,0.698774277295606,1.17282674302192));
#17162=CARTESIAN_POINT('Ctrl Pts',(-1.6865,0.653734345483144,1.20412620058719));
#17163=CARTESIAN_POINT('Ctrl Pts',(-1.6865,0.607002895401327,1.23271172365974));
#17164=CARTESIAN_POINT('Ctrl Pts',(-1.6865,0.559252531102573,1.26192051427065));
#17165=CARTESIAN_POINT('Ctrl Pts',(-1.6865,0.50973534369957,1.28829637345923));
#17166=CARTESIAN_POINT('Ctrl Pts',(-1.6865,0.45876129133789,1.31175582276503));
#17167=CARTESIAN_POINT('Ctrl Pts',(-1.6865,0.430153328292115,1.32492187544713));
#17168=CARTESIAN_POINT('Ctrl Pts',(-1.6865,0.401085755513973,1.33716870507987));
#17169=CARTESIAN_POINT('Ctrl Pts',(-1.6865,0.37160881565879,1.34847609048941));
#17170=CARTESIAN_POINT('Ctrl Pts',(-1.6865,0.351783551682333,1.35608108278946));
#17171=CARTESIAN_POINT('Ctrl Pts',(-1.6865,0.331773048043608,1.36326103519375));
#17172=CARTESIAN_POINT('Ctrl Pts',(-1.6865,0.311591988507046,1.37000865843416));
#17173=CARTESIAN_POINT('Ctrl Pts',(-1.6865,0.296897647160957,1.37492177407063));
#17174=CARTESIAN_POINT('Ctrl Pts',(-1.6865,0.282106107519082,1.37960750309936));
#17175=CARTESIAN_POINT('Ctrl Pts',(-1.6865,0.267259363096465,1.38405235084035));
#17176=CARTESIAN_POINT('Ctrl Pts',(-1.6865,0.211486458549836,1.40074975343081));
#17177=CARTESIAN_POINT('Ctrl Pts',(-1.6865,0.154865348764943,1.41407827312293));
#17178=CARTESIAN_POINT('Ctrl Pts',(-1.6865,0.0977297285868856,1.42396068228593));
#17179=CARTESIAN_POINT('Ctrl Pts',(-1.6865,0.0383682737208729,1.43422808086617));
#17180=CARTESIAN_POINT('Ctrl Pts',(-1.6865,-0.0215495424099283,1.4407765896995));
#17181=CARTESIAN_POINT('Ctrl Pts',(-1.6865,-0.0816809005958121,1.44346955384022));
#17182=CARTESIAN_POINT('Ctrl Pts',(-1.6865,-0.138204235749947,1.44600093379366));
#17183=CARTESIAN_POINT('Ctrl Pts',(-1.6865,-0.194917405599328,1.44512562109251));
#17184=CARTESIAN_POINT('Ctrl Pts',(-1.6865,-0.25154665254263,1.44068090653038));
#17185=CARTESIAN_POINT('Ctrl Pts',(-1.6865,-0.255161436183491,1.44039718950508));
#17186=CARTESIAN_POINT('Ctrl Pts',(-1.6865,-0.258775878501556,1.44009891087668));
#17187=CARTESIAN_POINT('Ctrl Pts',(-1.6865,-0.26238990830909,1.43978602091337));
#17188=CARTESIAN_POINT('',(-1.6865,-1.4635,-1.79227059055215E-16));
#17189=CARTESIAN_POINT('Origin',(-1.6865,0.,0.));
#17190=CARTESIAN_POINT('',(-1.6865,-1.29040238558681,0.694864466152488));
#17191=CARTESIAN_POINT('Origin',(-1.6865,0.,0.));
#17192=CARTESIAN_POINT('Ctrl Pts',(-1.6865,-1.2904023855868,0.694864466152506));
#17193=CARTESIAN_POINT('Ctrl Pts',(-1.6865,-1.30885072776436,0.651973324418185));
#17194=CARTESIAN_POINT('Ctrl Pts',(-1.6865,-1.32508620682539,0.608247465432293));
#17195=CARTESIAN_POINT('Ctrl Pts',(-1.6865,-1.33896629703696,0.563783087832447));
#17196=CARTESIAN_POINT('Ctrl Pts',(-1.6865,-1.35596322182967,0.509334040996302));
#17197=CARTESIAN_POINT('Ctrl Pts',(-1.6865,-1.36942928069231,0.453776801997275));
#17198=CARTESIAN_POINT('Ctrl Pts',(-1.6865,-1.37942205624868,0.397441414603066));
#17199=CARTESIAN_POINT('Ctrl Pts',(-1.6865,-1.38232583274047,0.381071050568741));
#17200=CARTESIAN_POINT('Ctrl Pts',(-1.6865,-1.38493600923725,0.364635008432255));
#17201=CARTESIAN_POINT('Ctrl Pts',(-1.6865,-1.38725324896998,0.34814152080314));
#17202=CARTESIAN_POINT('Ctrl Pts',(-1.6865,-1.38960490215389,0.331403087507239));
#17203=CARTESIAN_POINT('Ctrl Pts',(-1.6865,-1.39165518732054,0.314600489882574));
#17204=CARTESIAN_POINT('Ctrl Pts',(-1.6865,-1.39340187668387,0.29777267933919));
#17205=CARTESIAN_POINT('Ctrl Pts',(-1.6865,-1.39934087814592,0.240555641485509));
#17206=CARTESIAN_POINT('Ctrl Pts',(-1.6865,-1.40178440679026,0.182987687587848));
#17207=CARTESIAN_POINT('Ctrl Pts',(-1.6865,-1.40079973123309,0.125409327587869));
#17208=CARTESIAN_POINT('Ctrl Pts',(-1.6865,-1.40013542640393,0.0865644691722947));
#17209=CARTESIAN_POINT('Ctrl Pts',(-1.6865,-1.39790967150014,0.047714876544446));
#17210=CARTESIAN_POINT('Ctrl Pts',(-1.6865,-1.39413032699431,0.00896907191044844));
#17211=CARTESIAN_POINT('Ctrl Pts',(-1.6865,-1.3924216166484,-0.00854861062335397));
#17212=CARTESIAN_POINT('Ctrl Pts',(-1.6865,-1.39039520209046,-0.0260450144637056));
#17213=CARTESIAN_POINT('Ctrl Pts',(-1.6865,-1.38805116691589,-0.0435097336037873));
#17214=CARTESIAN_POINT('Ctrl Pts',(-1.6865,-1.38659889452283,-0.0543301895998504));
#17215=CARTESIAN_POINT('Ctrl Pts',(-1.6865,-1.38502456181393,-0.0651386374936669));
#17216=CARTESIAN_POINT('Ctrl Pts',(-1.6865,-1.38333070427925,-0.075918112300396));
#17217=CARTESIAN_POINT('Ctrl Pts',(-1.6865,-1.3745984754921,-0.131488807173018));
#17218=CARTESIAN_POINT('Ctrl Pts',(-1.6865,-1.36268151203973,-0.186387190848527));
#17219=CARTESIAN_POINT('Ctrl Pts',(-1.6865,-1.34763859383464,-0.24029577530626));
#17220=CARTESIAN_POINT('Ctrl Pts',(-1.6865,-1.33296240556968,-0.292890127267258));
#17221=CARTESIAN_POINT('Ctrl Pts',(-1.6865,-1.31531029836967,-0.344543270611425));
#17222=CARTESIAN_POINT('Ctrl Pts',(-1.6865,-1.29469447197158,-0.39493657110514));
#17223=CARTESIAN_POINT('Ctrl Pts',(-1.6865,-1.28220200568538,-0.425473140210423));
#17224=CARTESIAN_POINT('Ctrl Pts',(-1.6865,-1.26862049403763,-0.455546579887635));
#17225=CARTESIAN_POINT('Ctrl Pts',(-1.6865,-1.25394594681483,-0.485079483421535));
#17226=CARTESIAN_POINT('Ctrl Pts',(-1.6865,-1.24672102839584,-0.499619817475368));
#17227=CARTESIAN_POINT('Ctrl Pts',(-1.6865,-1.2392310819698,-0.51402903840633));
#17228=CARTESIAN_POINT('Ctrl Pts',(-1.6865,-1.2314752167513,-0.528297362306323));
#17229=CARTESIAN_POINT('Ctrl Pts',(-1.6865,-1.2265591600616,-0.537341342208399));
#17230=CARTESIAN_POINT('Ctrl Pts',(-1.6865,-1.22153530521596,-0.546330365042694));
#17231=CARTESIAN_POINT('Ctrl Pts',(-1.6865,-1.216406396493,-0.555256606025037));
#17232=CARTESIAN_POINT('Ctrl Pts',(-1.6865,-1.19005780148628,-0.601113126637944));
#17233=CARTESIAN_POINT('Ctrl Pts',(-1.6865,-1.16104088129756,-0.645141987000547));
#17234=CARTESIAN_POINT('Ctrl Pts',(-1.6865,-1.12937946594324,-0.687054969399394));
#17235=CARTESIAN_POINT('Ctrl Pts',(-1.6865,-1.11768049850354,-0.702541914973292));
#17236=CARTESIAN_POINT('Ctrl Pts',(-1.6865,-1.1056200916295,-0.717739646605471));
#17237=CARTESIAN_POINT('Ctrl Pts',(-1.6865,-1.09319816065634,-0.732632329346327));
#17238=CARTESIAN_POINT('Ctrl Pts',(-1.6865,-1.05946030810074,-0.773080721432396));
#17239=CARTESIAN_POINT('Ctrl Pts',(-1.6865,-1.02305711561143,-0.811282018446671));
#17240=CARTESIAN_POINT('Ctrl Pts',(-1.6865,-0.984269503995115,-0.847108021494535));
#17241=CARTESIAN_POINT('Ctrl Pts',(-1.6865,-0.966400601050763,-0.863612553345551));
#17242=CARTESIAN_POINT('Ctrl Pts',(-1.6865,-0.948025344634025,-0.87961236447309));
#17243=CARTESIAN_POINT('Ctrl Pts',(-1.6865,-0.929170102459808,-0.895091662773315));
#17244=CARTESIAN_POINT('Ctrl Pts',(-1.6865,-0.915705894475452,-0.906145166612746));
#17245=CARTESIAN_POINT('Ctrl Pts',(-1.6865,-0.90199692206211,-0.916933210091794));
#17246=CARTESIAN_POINT('Ctrl Pts',(-1.6865,-0.888052703846498,-0.927449361680719));
#17247=CARTESIAN_POINT('Ctrl Pts',(-1.6865,-0.879943703448156,-0.933564833778548));
#17248=CARTESIAN_POINT('Ctrl Pts',(-1.6865,-0.871762069645838,-0.939583081642751));
#17249=CARTESIAN_POINT('Ctrl Pts',(-1.6865,-0.863513813439513,-0.945500676396998));
#17250=CARTESIAN_POINT('Ctrl Pts',(-1.6865,-0.820858663551776,-0.976103010381695));
#17251=CARTESIAN_POINT('Ctrl Pts',(-1.6865,-0.776391161968852,-1.00404189628927));
#17252=CARTESIAN_POINT('Ctrl Pts',(-1.6865,-0.730402963290917,-1.02921107378108));
#17253=CARTESIAN_POINT('Ctrl Pts',(-1.6865,-0.684629141529403,-1.05426292354938));
#17254=CARTESIAN_POINT('Ctrl Pts',(-1.6865,-0.637347598234742,-1.07657108217632));
#17255=CARTESIAN_POINT('Ctrl Pts',(-1.6865,-0.588833516322352,-1.09598122749975));
#17256=CARTESIAN_POINT('Ctrl Pts',(-1.6865,-0.564550715329474,-1.10569660657222));
#17257=CARTESIAN_POINT('Ctrl Pts',(-1.6865,-0.539959039562968,-1.1146851418401));
#17258=CARTESIAN_POINT('Ctrl Pts',(-1.6865,-0.515093195527775,-1.1229224840706));
#17259=CARTESIAN_POINT('Ctrl Pts',(-1.6865,-0.496768718082754,-1.12899285882626));
#17260=CARTESIAN_POINT('Ctrl Pts',(-1.6865,-0.478295351359644,-1.13465521308558));
#17261=CARTESIAN_POINT('Ctrl Pts',(-1.6865,-0.45968725369228,-1.13989858657083));
#17262=CARTESIAN_POINT('Ctrl Pts',(-1.6865,-0.450689443834044,-1.1424339815628));
#17263=CARTESIAN_POINT('Ctrl Pts',(-1.6865,-0.441661083642265,-1.14487103249921));
#17264=CARTESIAN_POINT('Ctrl Pts',(-1.6865,-0.432616279421598,-1.1472055526786));
#17265=CARTESIAN_POINT('Ctrl Pts',(-1.6865,-0.383781112234802,-1.15981021282161));
#17266=CARTESIAN_POINT('Ctrl Pts',(-1.6865,-0.334370220207706,-1.16945779617145));
#17267=CARTESIAN_POINT('Ctrl Pts',(-1.6865,-0.284637624516386,-1.17602215875609));
#17268=CARTESIAN_POINT('Ctrl Pts',(-1.6865,-0.235926324583538,-1.18245171728372));
#17269=CARTESIAN_POINT('Ctrl Pts',(-1.6865,-0.186905453024311,-1.18592341187249));
#17270=CARTESIAN_POINT('Ctrl Pts',(-1.6865,-0.137820117989715,-1.18626955672358));
#17271=CARTESIAN_POINT('Ctrl Pts',(-1.6865,-0.0887347829551201,-1.18661570157467));
#17272=CARTESIAN_POINT('Ctrl Pts',(-1.6865,-0.0395840767290218,-1.18383647660889));
#17273=CARTESIAN_POINT('Ctrl Pts',(-1.6865,0.00936663037056407,-1.17771275306651));
#17274=CARTESIAN_POINT('Ctrl Pts',(-7.90147783942094,-0.510216505388438,
1.06149619882937));
#17275=CARTESIAN_POINT('Ctrl Pts',(-7.87525430423351,-0.860016296466908,
0.89336217518757));
#17276=CARTESIAN_POINT('Ctrl Pts',(-7.82280723385865,-1.37476509314629,
0.187438301404127));
#17277=CARTESIAN_POINT('Ctrl Pts',(-7.74413662829635,-0.911603039763577,
-1.0476379059846));
#17278=CARTESIAN_POINT('Ctrl Pts',(-7.66546602273408,0.37338601803043,-1.33626108168095));
#17279=CARTESIAN_POINT('Ctrl Pts',(-7.58679541717176,1.32164391460705,-0.423509280609249));
#17280=CARTESIAN_POINT('Ctrl Pts',(-7.50812481160949,1.08034427095369,0.871377146278108));
#17281=CARTESIAN_POINT('Ctrl Pts',(-7.42945420604718,-0.133733706588163,
1.38132579741601));
#17282=CARTESIAN_POINT('Ctrl Pts',(-7.3507836004849,-1.22732977726997,0.647920010724189));
#17283=CARTESIAN_POINT('Ctrl Pts',(-7.27211299492261,-1.2160203437836,-0.668923549344045));
#17284=CARTESIAN_POINT('Ctrl Pts',(-7.19344238936034,-0.109920457047265,
-1.38347881456886));
#17285=CARTESIAN_POINT('Ctrl Pts',(-7.11477178379802,1.095127328248,-0.852540070304724));
#17286=CARTESIAN_POINT('Ctrl Pts',(-7.03610117823576,1.31425240912282,0.445947499710114));
#17287=CARTESIAN_POINT('Ctrl Pts',(-6.95743057267344,0.350169610287078,
1.34294482869753));
#17288=CARTESIAN_POINT('Ctrl Pts',(-6.87875996711116,-0.929164632477942,
1.03091115994185));
#17289=CARTESIAN_POINT('Ctrl Pts',(-6.80008936154887,-1.37198482640854,
-0.209241177774123));
#17290=CARTESIAN_POINT('Ctrl Pts',(-6.72141875598658,-0.579624239257938,
-1.26101500289363));
#17291=CARTESIAN_POINT('Ctrl Pts',(-6.64274815042429,0.734564342461029,
-1.17751395698303));
#17292=CARTESIAN_POINT('Ctrl Pts',(-6.564077544862,1.38743422631486,-0.0339118586638691));
#17293=CARTESIAN_POINT('Ctrl Pts',(-6.4854069392997,0.791214847056285,1.14022045088028));
#17294=CARTESIAN_POINT('Ctrl Pts',(-6.40673633373742,-0.517325047723218,
1.28782705533921));
#17295=CARTESIAN_POINT('Ctrl Pts',(-6.32806572817513,-1.36012387380599,
0.276019467196043));
#17296=CARTESIAN_POINT('Ctrl Pts',(-6.24939512261283,-0.978420656071388,
-0.984284868996692));
#17297=CARTESIAN_POINT('Ctrl Pts',(-6.17072451705056,0.284142091338451,
-1.35845020984985));
#17298=CARTESIAN_POINT('Ctrl Pts',(-6.09205391148824,1.29089537055166,-0.509620287250948));
#17299=CARTESIAN_POINT('Ctrl Pts',(-6.01338330592598,1.13547214593956,0.798014222500227));
#17300=CARTESIAN_POINT('Ctrl Pts',(-5.93471270036367,-0.0422020497217742,
1.38720679169256));
#17301=CARTESIAN_POINT('Ctrl Pts',(-5.85604209480139,-1.181882283109,0.727514923408978));
#17302=CARTESIAN_POINT('Ctrl Pts',(-5.77737148923909,-1.25752909475175,
-0.587149274616201));
#17303=CARTESIAN_POINT('Ctrl Pts',(-5.69870088367681,-0.201038633207167,
-1.37321053124158));
#17304=CARTESIAN_POINT('Ctrl Pts',(-5.62003027811452,1.03644432469548,-0.922988004686612));
#17305=CARTESIAN_POINT('Ctrl Pts',(-5.54135967255223,1.34082978479473,0.358188753595292));
#17306=CARTESIAN_POINT('Ctrl Pts',(-5.46268906698994,0.438083431536926,
1.31689278305031));
#17307=CARTESIAN_POINT('Ctrl Pts',(-5.38401846142764,-0.859063801779334,
1.09001517396937));
#17308=CARTESIAN_POINT('Ctrl Pts',(-5.30534785586536,-1.38280694114473,
-0.118189079598716));
#17309=CARTESIAN_POINT('Ctrl Pts',(-5.22667725030306,-0.66162677306598,
-1.21998922461717));
#17310=CARTESIAN_POINT('Ctrl Pts',(-5.14800664474078,0.655207470874117,
-1.22344875868442));
#17311=CARTESIAN_POINT('Ctrl Pts',(-5.06933603917847,1.38216685417029,-0.12545310777169));
#17312=CARTESIAN_POINT('Ctrl Pts',(-4.9906654336162,0.86477919209241,1.08548636285362));
#17313=CARTESIAN_POINT('Ctrl Pts',(-4.9119948280539,-0.431158056335988,
1.31917641938943));
#17314=CARTESIAN_POINT('Ctrl Pts',(-4.83332422249162,-1.33892925095376,
0.365228908983454));
#17315=CARTESIAN_POINT('Ctrl Pts',(-4.75465361692932,-1.04127965837587,
-0.917529491661948));
#17316=CARTESIAN_POINT('Ctrl Pts',(-4.67598301136704,0.193820620708426,
-1.37424788957624));
#17317=CARTESIAN_POINT('Ctrl Pts',(-4.59731240580474,1.25442668732974,-0.593748584109574));
#17318=CARTESIAN_POINT('Ctrl Pts',(-4.51864180024246,1.18568853815801,0.721294936553209));
#17319=CARTESIAN_POINT('Ctrl Pts',(-4.43997119468016,0.049490244982279,
1.38696590104707));
#17320=CARTESIAN_POINT('Ctrl Pts',(-4.36130058911787,-1.13126347935192,
0.803969299976234));
#17321=CARTESIAN_POINT('Ctrl Pts',(-4.28262998355558,-1.29355524026402,
-0.502830523536472));
#17322=CARTESIAN_POINT('Ctrl Pts',(-4.20395937799329,-0.29127585234018,
-1.35693849265711));
#17323=CARTESIAN_POINT('Ctrl Pts',(-4.125288772431,0.973235439907126,-0.989412185868934));
#17324=CARTESIAN_POINT('Ctrl Pts',(-4.04661816686871,1.36155538052876,0.268869188915402));
#17325=CARTESIAN_POINT('Ctrl Pts',(-3.96794756130642,0.524084520485498,
1.28509109030307));
#17326=CARTESIAN_POINT('Ctrl Pts',(-3.88927695574413,-0.785212894157578,
1.14436200828378));
#17327=CARTESIAN_POINT('Ctrl Pts',(-3.81060635018184,-1.38759323720175,
-0.0266214744418142));
#17328=CARTESIAN_POINT('Ctrl Pts',(-3.73193574461955,-0.740741232249389,
-1.17363798581818));
#17329=CARTESIAN_POINT('Ctrl Pts',(-3.65326513905726,0.572990579286003,
-1.26404331095425));
#17330=CARTESIAN_POINT('Ctrl Pts',(-3.57459453349497,1.3708663395606,-0.216446696849244));
#17331=CARTESIAN_POINT('Ctrl Pts',(-3.49592392793268,0.934568764120381,
1.02601409348018));
#17332=CARTESIAN_POINT('Ctrl Pts',(-3.41725332237039,-0.34310905511451,
1.34476759219195));
#17333=CARTESIAN_POINT('Ctrl Pts',(-3.3385827168081,-1.31189019805787,0.452844114240954));
#17334=CARTESIAN_POINT('Ctrl Pts',(-3.25991211124581,-1.09959347693818,
-0.846769085313812));
#17335=CARTESIAN_POINT('Ctrl Pts',(-3.18124150568352,0.102653133571944,
-1.38404698750922));
#17336=CARTESIAN_POINT('Ctrl Pts',(-3.10257090012123,1.2124824062959,-0.675285143647363));
#17337=CARTESIAN_POINT('Ctrl Pts',(-3.02390029455893,1.23072943933634,0.641427153820911));
#17338=CARTESIAN_POINT('Ctrl Pts',(-2.94522968899665,0.140966433426828,
1.38067098062933));
#17339=CARTESIAN_POINT('Ctrl Pts',(-2.86655908343435,-1.07570655288296,
0.876914196682235));
#17340=CARTESIAN_POINT('Ctrl Pts',(-2.78788847787207,-1.32393530813497,
-0.416316627394508));
#17341=CARTESIAN_POINT('Ctrl Pts',(-2.70921787230977,-0.38024109152726,
-1.33474396280885));
#17342=CARTESIAN_POINT('Ctrl Pts',(-2.63054726674748,0.905777314237609,
-1.05151653620214));
#17343=CARTESIAN_POINT('Ctrl Pts',(-2.5518766611852,1.37633981097026,0.178374023112081));
#17344=CARTESIAN_POINT('Ctrl Pts',(-2.4732060556229,0.607794121628612,1.24768375090184));
#17345=CARTESIAN_POINT('Ctrl Pts',(-2.39453545006062,-0.707927190944584,
1.19370650897096));
#17346=CARTESIAN_POINT('Ctrl Pts',(-2.31586484449832,-1.38633664878164,
0.0650760140720061));
#17347=CARTESIAN_POINT('Ctrl Pts',(-2.23719423893603,-0.81659578676643,
-1.12218984289901));
#17348=CARTESIAN_POINT('Ctrl Pts',(-2.15852363337374,0.488222034063068,
-1.29907078650092));
#17349=CARTESIAN_POINT('Ctrl Pts',(-2.07985302781145,1.35367817671458,-0.306589740084279));
#17350=CARTESIAN_POINT('Ctrl Pts',(-2.00118242224916,1.00009581383204,0.962242750523822));
#17351=CARTESIAN_POINT('Ctrl Pts',(-1.92251181668687,-0.253212907927416,
1.36414589400647));
#17352=CARTESIAN_POINT('Ctrl Pts',(-1.84384121112458,-1.2797987521583,0.539147881509388));
#17353=CARTESIAN_POINT('Ctrl Pts',(-1.76517060556229,-1.1517468612252,-0.773686852560318));
#17354=CARTESIAN_POINT('Ctrl Pts',(-1.71272353518743,-0.378730543625381,
-1.1807993824396));
#17355=CARTESIAN_POINT('Ctrl Pts',(-1.6865,0.00936663037056419,-1.17771275306651));
#17356=CARTESIAN_POINT('Ctrl Pts',(-7.84648522628062,-0.551480035117362,
1.14734422509853));
#17357=CARTESIAN_POINT('Ctrl Pts',(-7.82026169109319,-0.929569726514428,
0.965612438135244));
#17358=CARTESIAN_POINT('Ctrl Pts',(-7.76781462071833,-1.48594859993651,
0.202597289482033));
#17359=CARTESIAN_POINT('Ctrl Pts',(-7.68914401515604,-0.985328524405893,
-1.13236514907102));
#17360=CARTESIAN_POINT('Ctrl Pts',(-7.61047340959375,0.403583443814669,
-1.444330593912));
#17361=CARTESIAN_POINT('Ctrl Pts',(-7.53180280403146,1.42853127004439,-0.457760402645369));
#17362=CARTESIAN_POINT('Ctrl Pts',(-7.45313219846917,1.16771662655407,0.941849379929546));
#17363=CARTESIAN_POINT('Ctrl Pts',(-7.37446159290689,-0.144549359784947,
1.4930398982047));
#17364=CARTESIAN_POINT('Ctrl Pts',(-7.29579098734458,-1.32658951939263,
0.700320249332966));
#17365=CARTESIAN_POINT('Ctrl Pts',(-7.21712038178231,-1.31436544057442,
-0.72302243966458));
#17366=CARTESIAN_POINT('Ctrl Pts',(-7.13844977622001,-0.118810224428935,
-1.49536703964862));
#17367=CARTESIAN_POINT('Ctrl Pts',(-7.05977917065772,1.18369525693882,-0.921488863933704));
#17368=CARTESIAN_POINT('Ctrl Pts',(-6.98110856509543,1.42054197988822,0.482013302594748));
#17369=CARTESIAN_POINT('Ctrl Pts',(-6.90243795953314,0.378489419567362,
1.45155488595369));
#17370=CARTESIAN_POINT('Ctrl Pts',(-6.82376735397085,-1.00431040300948,
1.11428563498703));
#17371=CARTESIAN_POINT('Ctrl Pts',(-6.74509674840856,-1.48294348038045,
-0.22616346364377));
#17372=CARTESIAN_POINT('Ctrl Pts',(-6.66642614284627,-0.62650108815569,
-1.36299902244414));
#17373=CARTESIAN_POINT('Ctrl Pts',(-6.58775553728398,0.79397190231618,-1.27274486711051));
#17374=CARTESIAN_POINT('Ctrl Pts',(-6.50908493172169,1.49964234353539,-0.0366544649366292));
#17375=CARTESIAN_POINT('Ctrl Pts',(-6.4304143261594,0.855203990917139,1.23243526552375));
#17376=CARTESIAN_POINT('Ctrl Pts',(-6.35174372059711,-0.559163477607003,
1.3919794875371));
#17377=CARTESIAN_POINT('Ctrl Pts',(-6.27307311503482,-1.4701232785863,0.298342417100889));
#17378=CARTESIAN_POINT('Ctrl Pts',(-6.19440250947252,-1.05754998529305,
-1.06388846379349));
#17379=CARTESIAN_POINT('Ctrl Pts',(-6.11573190391024,0.30712195480691,-1.46831425781266));
#17380=CARTESIAN_POINT('Ctrl Pts',(-6.03706129834795,1.39529595135832,-0.550835598106954));
#17381=CARTESIAN_POINT('Ctrl Pts',(-5.95839069278566,1.22730294356278,0.862553262783086));
#17382=CARTESIAN_POINT('Ctrl Pts',(-5.87972008722336,-0.0456151214568538,
1.49939651524061));
#17383=CARTESIAN_POINT('Ctrl Pts',(-5.80104948166107,-1.27746647964148,
0.786352364678105));
#17384=CARTESIAN_POINT('Ctrl Pts',(-5.72237887609879,-1.35923119305369,
-0.634634707354204));
#17385=CARTESIAN_POINT('Ctrl Pts',(-5.64370827053649,-0.217297541984914,
-1.48426831353898));
#17386=CARTESIAN_POINT('Ctrl Pts',(-5.56503766497421,1.12026629194425,-0.99763424323164));
#17387=CARTESIAN_POINT('Ctrl Pts',(-5.48636705941191,1.44926878882929,0.3871571074734));
#17388=CARTESIAN_POINT('Ctrl Pts',(-5.40769645384962,0.473513231455331,
1.4233958928661));
#17389=CARTESIAN_POINT('Ctrl Pts',(-5.32902584828733,-0.928540199248638,
1.17816965948887));
#17390=CARTESIAN_POINT('Ctrl Pts',(-5.25035524272504,-1.49464082876438,
-0.127747568099473));
#17391=CARTESIAN_POINT('Ctrl Pts',(-5.17168463716275,-0.715135539896414,
-1.31865530285515));
#17392=CARTESIAN_POINT('Ctrl Pts',(-5.09301403160046,0.708197079535336,
-1.3223946251796));
#17393=CARTESIAN_POINT('Ctrl Pts',(-5.01434342603817,1.4939489750446,-0.135599071274354));
#17394=CARTESIAN_POINT('Ctrl Pts',(-4.93567282047588,0.934717819175246,
1.17327458281694));
#17395=CARTESIAN_POINT('Ctrl Pts',(-4.85700221491359,-0.466027769658844,
1.42586421726407));
#17396=CARTESIAN_POINT('Ctrl Pts',(-4.7783316093513,-1.4472145501712,0.39476663225298));
#17397=CARTESIAN_POINT('Ctrl Pts',(-4.69966100378902,-1.12549268105498,
-0.991734275428277));
#17398=CARTESIAN_POINT('Ctrl Pts',(-4.62099039822671,0.209495775981166,
-1.48538956776103));
#17399=CARTESIAN_POINT('Ctrl Pts',(-4.54231979266444,1.35587787983082,-0.641767733026107));
#17400=CARTESIAN_POINT('Ctrl Pts',(-4.46364918710213,1.28158056385069,0.779629339191021));
#17401=CARTESIAN_POINT('Ctrl Pts',(-4.38497858153985,0.0534927462215688,
1.49913614267282));
#17402=CARTESIAN_POINT('Ctrl Pts',(-4.30630797597756,-1.22275390296327,
0.868989954463811));
#17403=CARTESIAN_POINT('Ctrl Pts',(-4.22763737041526,-1.39817093683387,
-0.543496715314725));
#17404=CARTESIAN_POINT('Ctrl Pts',(-4.14896676485299,-0.314832655511832,
-1.46668028117384));
#17405=CARTESIAN_POINT('Ctrl Pts',(-4.07029615929068,1.05194541711039,-1.069430450105));
#17406=CARTESIAN_POINT('Ctrl Pts',(-3.9916255537284,1.47167055776957,0.290613863289574));
#17407=CARTESIAN_POINT('Ctrl Pts',(-3.91295494816611,0.566469619679939,
1.38902225256277));
#17408=CARTESIAN_POINT('Ctrl Pts',(-3.83428434260381,-0.848716632785046,
1.23691176951412));
#17409=CARTESIAN_POINT('Ctrl Pts',(-3.75561373704153,-1.49981421435604,
-0.0287744741790862));
#17410=CARTESIAN_POINT('Ctrl Pts',(-3.67694313147923,-0.800648345279968,
-1.26855542852604));
#17411=CARTESIAN_POINT('Ctrl Pts',(-3.59827252591695,0.619330933925767,
-1.36627224355318));
#17412=CARTESIAN_POINT('Ctrl Pts',(-3.51960192035466,1.4817345364132,-0.2339517258239));
#17413=CARTESIAN_POINT('Ctrl Pts',(-3.44093131479236,1.01015159136086,1.10899252048419));
#17414=CARTESIAN_POINT('Ctrl Pts',(-3.36226070923008,-0.370857845180013,
1.45352506462352));
#17415=CARTESIAN_POINT('Ctrl Pts',(-3.28359010366778,-1.41798872606892,
0.489467677714918));
#17416=CARTESIAN_POINT('Ctrl Pts',(-3.2049194981055,-1.18852260338978,-0.915251153134768));
#17417=CARTESIAN_POINT('Ctrl Pts',(-3.1262488925432,0.110955159445615,-1.49598116331925));
#17418=CARTESIAN_POINT('Ctrl Pts',(-3.04757828698092,1.31054137398826,-0.729898525037658));
#17419=CARTESIAN_POINT('Ctrl Pts',(-2.96890768141862,1.33026412759513,0.693302285556365));
#17420=CARTESIAN_POINT('Ctrl Pts',(-2.89023707585633,0.152367030144226,
1.49233212340576));
#17421=CARTESIAN_POINT('Ctrl Pts',(-2.81156647029404,-1.1627038351263,0.947834236787512));
#17422=CARTESIAN_POINT('Ctrl Pts',(-2.73289586473176,-1.43100797899029,
-0.449986046846273));
#17423=CARTESIAN_POINT('Ctrl Pts',(-2.65422525916946,-0.410992918288442,
-1.44269077873544));
#17424=CARTESIAN_POINT('Ctrl Pts',(-2.57555465360718,0.979031645955821,
-1.13655746175787));
#17425=CARTESIAN_POINT('Ctrl Pts',(-2.49688404804488,1.48765067235418,0.192799941771742));
#17426=CARTESIAN_POINT('Ctrl Pts',(-2.41821344248259,0.65694919705645,1.34858961146087));
#17427=CARTESIAN_POINT('Ctrl Pts',(-2.3395428369203,-0.765180483186115,
1.29024698443646));
#17428=CARTESIAN_POINT('Ctrl Pts',(-2.26087223135801,-1.49845599991427,
0.0703390073561241));
#17429=CARTESIAN_POINT('Ctrl Pts',(-2.18220162579572,-0.882637602677711,
-1.21294644025509));
#17430=CARTESIAN_POINT('Ctrl Pts',(-2.10353102023343,0.52770677084464,-1.40413255038478));
#17431=CARTESIAN_POINT('Ctrl Pts',(-2.02486041467114,1.4631562886501,-0.33138504701957));
#17432=CARTESIAN_POINT('Ctrl Pts',(-1.94618980910885,1.08097811166053,1.04006369893171));
#17433=CARTESIAN_POINT('Ctrl Pts',(-1.86751920354656,-0.273691387638793,
1.47447057785628));
#17434=CARTESIAN_POINT('Ctrl Pts',(-1.78884859798427,-1.38330189895777,
0.582751223231977));
#17435=CARTESIAN_POINT('Ctrl Pts',(-1.71017799242198,-1.24489386910607,
-0.836258427772682));
#17436=CARTESIAN_POINT('Ctrl Pts',(-1.65773092204712,-0.409360205506362,
-1.27629599986891));
#17437=CARTESIAN_POINT('Ctrl Pts',(-1.63150738685969,0.0101241523767517,
-1.27295974073757));
#17438=CARTESIAN_POINT('Ctrl Pts',(-7.79149261314031,-0.592743564846287,
1.23319225136769));
#17439=CARTESIAN_POINT('Ctrl Pts',(-7.76526907795288,-0.999123156561948,
1.03786270108292));
#17440=CARTESIAN_POINT('Ctrl Pts',(-7.71282200757802,-1.59713210672673,
0.21775627755994));
#17441=CARTESIAN_POINT('Ctrl Pts',(-7.63415140201573,-1.05905400904821,
-1.21709239215744));
#17442=CARTESIAN_POINT('Ctrl Pts',(-7.55548079645344,0.433780869598909,
-1.55240010614304));
#17443=CARTESIAN_POINT('Ctrl Pts',(-7.47681019089115,1.53541862548172,-0.492011524681491));
#17444=CARTESIAN_POINT('Ctrl Pts',(-7.39813958532886,1.25508898215445,1.01232161358098));
#17445=CARTESIAN_POINT('Ctrl Pts',(-7.31946897976657,-0.155365012981731,
1.60475399899339));
#17446=CARTESIAN_POINT('Ctrl Pts',(-7.24079837420427,-1.42584926151528,
0.752720487941745));
#17447=CARTESIAN_POINT('Ctrl Pts',(-7.16212776864199,-1.41271053736525,
-0.777121329985117));
#17448=CARTESIAN_POINT('Ctrl Pts',(-7.08345716307969,-0.127699991810606,
-1.60725526472837));
#17449=CARTESIAN_POINT('Ctrl Pts',(-7.00478655751741,1.27226318562964,-0.990437657562687));
#17450=CARTESIAN_POINT('Ctrl Pts',(-6.92611595195512,1.52683155065362,0.518079105479383));
#17451=CARTESIAN_POINT('Ctrl Pts',(-6.84744534639283,0.406809228847646,
1.56016494320984));
#17452=CARTESIAN_POINT('Ctrl Pts',(-6.76877474083054,-1.07945617354101,
1.19766011003222));
#17453=CARTESIAN_POINT('Ctrl Pts',(-6.69010413526824,-1.59390213435235,
-0.243085749513416));
#17454=CARTESIAN_POINT('Ctrl Pts',(-6.61143352970597,-0.673377937053443,
-1.46498304199465));
#17455=CARTESIAN_POINT('Ctrl Pts',(-6.53276292414366,0.853379462171331,
-1.36797577723799));
#17456=CARTESIAN_POINT('Ctrl Pts',(-6.45409231858138,1.61185046075593,-0.0393970712093886));
#17457=CARTESIAN_POINT('Ctrl Pts',(-6.37542171301908,0.919193134777992,
1.32465008016721));
#17458=CARTESIAN_POINT('Ctrl Pts',(-6.2967511074568,-0.601001907490788,
1.49613191973499));
#17459=CARTESIAN_POINT('Ctrl Pts',(-6.2180805018945,-1.58012268336662,0.320665367005734));
#17460=CARTESIAN_POINT('Ctrl Pts',(-6.13940989633221,-1.1366793145147,-1.14349205859028));
#17461=CARTESIAN_POINT('Ctrl Pts',(-6.06073929076993,0.330101818275368,
-1.57817830577548));
#17462=CARTESIAN_POINT('Ctrl Pts',(-5.98206868520763,1.49969653216498,-0.592050908962961));
#17463=CARTESIAN_POINT('Ctrl Pts',(-5.90339807964535,1.319133741186,0.927092303065946));
#17464=CARTESIAN_POINT('Ctrl Pts',(-5.82472747408305,-0.0490281931919314,
1.61158623878866));
#17465=CARTESIAN_POINT('Ctrl Pts',(-5.74605686852077,-1.37305067617395,
0.845189805947231));
#17466=CARTESIAN_POINT('Ctrl Pts',(-5.66738626295846,-1.46093329135563,
-0.682120140092207));
#17467=CARTESIAN_POINT('Ctrl Pts',(-5.5887156573962,-0.233556450762664,
-1.59532609583638));
#17468=CARTESIAN_POINT('Ctrl Pts',(-5.51004505183388,1.20408825919302,-1.07228048177667));
#17469=CARTESIAN_POINT('Ctrl Pts',(-5.43137444627161,1.55770779286385,0.416125461351507));
#17470=CARTESIAN_POINT('Ctrl Pts',(-5.35270384070931,0.508943031373735,
1.52989900268188));
#17471=CARTESIAN_POINT('Ctrl Pts',(-5.27403323514702,-0.998016596717941,
1.26632414500837));
#17472=CARTESIAN_POINT('Ctrl Pts',(-5.19536262958473,-1.60647471638402,
-0.13730605660023));
#17473=CARTESIAN_POINT('Ctrl Pts',(-5.11669202402244,-0.768644306726847,
-1.41732138109313));
#17474=CARTESIAN_POINT('Ctrl Pts',(-5.03802141846015,0.761186688196555,
-1.42134049167478));
#17475=CARTESIAN_POINT('Ctrl Pts',(-4.95935081289786,1.60573109591891,-0.145745034777019));
#17476=CARTESIAN_POINT('Ctrl Pts',(-4.88068020733557,1.00465644625808,1.26106280278026));
#17477=CARTESIAN_POINT('Ctrl Pts',(-4.80200960177328,-0.5008974829817,1.5325520151387));
#17478=CARTESIAN_POINT('Ctrl Pts',(-4.72333899621098,-1.55549984938864,
0.424304355522506));
#17479=CARTESIAN_POINT('Ctrl Pts',(-4.6446683906487,-1.20970570373407,-1.0659390591946));
#17480=CARTESIAN_POINT('Ctrl Pts',(-4.5659977850864,0.225170931253902,-1.59653124594583));
#17481=CARTESIAN_POINT('Ctrl Pts',(-4.48732717952412,1.45732907233191,-0.689786881942641));
#17482=CARTESIAN_POINT('Ctrl Pts',(-4.40865657396183,1.37747258954337,0.837963741828835));
#17483=CARTESIAN_POINT('Ctrl Pts',(-4.32998596839954,0.0574952474608585,
1.61130638429858));
#17484=CARTESIAN_POINT('Ctrl Pts',(-4.25131536283725,-1.31424432657462,
0.93401060895139));
#17485=CARTESIAN_POINT('Ctrl Pts',(-4.17264475727496,-1.50278663340373,
-0.584162907092979));
#17486=CARTESIAN_POINT('Ctrl Pts',(-4.09397415171267,-0.338389458683483,
-1.57642206969058));
#17487=CARTESIAN_POINT('Ctrl Pts',(-4.01530354615038,1.13065539431366,-1.14944871434106));
#17488=CARTESIAN_POINT('Ctrl Pts',(-3.93663294058808,1.58178573501038,0.312358537663747));
#17489=CARTESIAN_POINT('Ctrl Pts',(-3.85796233502579,0.608854718874381,
1.49295341482247));
#17490=CARTESIAN_POINT('Ctrl Pts',(-3.77929172946351,-0.912220371412514,
1.32946153074446));
#17491=CARTESIAN_POINT('Ctrl Pts',(-3.70062112390121,-1.61203519151034,
-0.0309274739163594));
#17492=CARTESIAN_POINT('Ctrl Pts',(-3.62195051833893,-0.860555458310546,
-1.36347287123389));
#17493=CARTESIAN_POINT('Ctrl Pts',(-3.54327991277663,0.665671288565531,
-1.46850117615212));
#17494=CARTESIAN_POINT('Ctrl Pts',(-3.46460930721435,1.59260273326579,-0.251456754798555));
#17495=CARTESIAN_POINT('Ctrl Pts',(-3.38593870165205,1.08573441860134,1.19197094748821));
#17496=CARTESIAN_POINT('Ctrl Pts',(-3.30726809608977,-0.398606635245517,
1.56228253705509));
#17497=CARTESIAN_POINT('Ctrl Pts',(-3.22859749052747,-1.52408725407996,
0.526091241188881));
#17498=CARTESIAN_POINT('Ctrl Pts',(-3.14992688496519,-1.27745172984138,
-0.983733220955725));
#17499=CARTESIAN_POINT('Ctrl Pts',(-3.07125627940289,0.119257185319287,
-1.60791533912927));
#17500=CARTESIAN_POINT('Ctrl Pts',(-2.99258567384061,1.40860034168063,-0.784511906427953));
#17501=CARTESIAN_POINT('Ctrl Pts',(-2.9139150682783,1.42979881585392,0.745177417291821));
#17502=CARTESIAN_POINT('Ctrl Pts',(-2.83524446271603,0.163767626861624,
1.60399326618219));
#17503=CARTESIAN_POINT('Ctrl Pts',(-2.75657385715372,-1.24970111736964,
1.01875427689279));
#17504=CARTESIAN_POINT('Ctrl Pts',(-2.67790325159145,-1.53808064984562,
-0.48365546629804));
#17505=CARTESIAN_POINT('Ctrl Pts',(-2.59923264602914,-0.441744745049623,
-1.55063759466203));
#17506=CARTESIAN_POINT('Ctrl Pts',(-2.52056204046686,1.05228597767403,-1.2215983873136));
#17507=CARTESIAN_POINT('Ctrl Pts',(-2.44189143490457,1.59896153373811,0.207225860431403));
#17508=CARTESIAN_POINT('Ctrl Pts',(-2.36322082934228,0.706104272484286,
1.4494954720199));
#17509=CARTESIAN_POINT('Ctrl Pts',(-2.28455022377999,-0.822433775427645,
1.38678745990196));
#17510=CARTESIAN_POINT('Ctrl Pts',(-2.2058796182177,-1.6105753510469,0.0756020006402417));
#17511=CARTESIAN_POINT('Ctrl Pts',(-2.12720901265541,-0.948679418588992,
-1.30370303761117));
#17512=CARTESIAN_POINT('Ctrl Pts',(-2.04853840709312,0.567191507626213,
-1.50919431426864));
#17513=CARTESIAN_POINT('Ctrl Pts',(-1.96986780153083,1.57263440058562,-0.35618035395486));
#17514=CARTESIAN_POINT('Ctrl Pts',(-1.89119719596854,1.16186040948903,1.11788464733959));
#17515=CARTESIAN_POINT('Ctrl Pts',(-1.81252659040625,-0.294169867350172,
1.58479526170609));
#17516=CARTESIAN_POINT('Ctrl Pts',(-1.73385598484396,-1.48680504575724,
0.626354564954566));
#17517=CARTESIAN_POINT('Ctrl Pts',(-1.65518537928167,-1.33804087698695,
-0.898830002985046));
#17518=CARTESIAN_POINT('Ctrl Pts',(-1.60273830890681,-0.439989867387345,
-1.37179261729822));
#17519=CARTESIAN_POINT('Ctrl Pts',(-1.57651477371938,0.0108816743829391,
-1.36820672840862));
#17520=CARTESIAN_POINT('Ctrl Pts',(-7.7365,-0.634007094575211,1.31904027763685));
#17521=CARTESIAN_POINT('Ctrl Pts',(-7.71027646481257,-1.06867658660947,
1.11011296403059));
#17522=CARTESIAN_POINT('Ctrl Pts',(-7.65782939443771,-1.70831561351695,
0.232915265637844));
#17523=CARTESIAN_POINT('Ctrl Pts',(-7.57915878887542,-1.13277949369053,
-1.30181963524385));
#17524=CARTESIAN_POINT('Ctrl Pts',(-7.50048818331312,0.463978295383148,
-1.66046961837409));
#17525=CARTESIAN_POINT('Ctrl Pts',(-7.42181757775084,1.64230598091905,-0.526262646717611));
#17526=CARTESIAN_POINT('Ctrl Pts',(-7.34314697218855,1.34246133775483,1.08279384723242));
#17527=CARTESIAN_POINT('Ctrl Pts',(-7.26447636662625,-0.166180666178515,
1.71646809978208));
#17528=CARTESIAN_POINT('Ctrl Pts',(-7.18580576106397,-1.52510900363794,
0.805120726550522));
#17529=CARTESIAN_POINT('Ctrl Pts',(-7.10713515550167,-1.51105563415607,
-0.831220220305652));
#17530=CARTESIAN_POINT('Ctrl Pts',(-7.0284645499394,-0.136589759192276,
-1.71914348980813));
#17531=CARTESIAN_POINT('Ctrl Pts',(-6.94979394437708,1.36083111432046,-1.05938645119167));
#17532=CARTESIAN_POINT('Ctrl Pts',(-6.87112333881482,1.63312112141902,0.554144908364018));
#17533=CARTESIAN_POINT('Ctrl Pts',(-6.7924527332525,0.43512903812793,1.668775000466));
#17534=CARTESIAN_POINT('Ctrl Pts',(-6.71378212769024,-1.15460194407255,
1.28103458507741));
#17535=CARTESIAN_POINT('Ctrl Pts',(-6.63511152212792,-1.70486078832426,
-0.260008035383061));
#17536=CARTESIAN_POINT('Ctrl Pts',(-6.55644091656565,-0.720254785951196,
-1.56696706154517));
#17537=CARTESIAN_POINT('Ctrl Pts',(-6.47777031100335,0.912787022026482,
-1.46320668736547));
#17538=CARTESIAN_POINT('Ctrl Pts',(-6.39909970544107,1.72405857797647,-0.0421396774821499));
#17539=CARTESIAN_POINT('Ctrl Pts',(-6.32042909987877,0.983182278638845,
1.41686489481067));
#17540=CARTESIAN_POINT('Ctrl Pts',(-6.24175849431648,-0.642840337374572,
1.60028435193288));
#17541=CARTESIAN_POINT('Ctrl Pts',(-6.1630878887542,-1.69012208814694,0.342988316910582));
#17542=CARTESIAN_POINT('Ctrl Pts',(-6.08441728319189,-1.21580864373636,
-1.22309565338708));
#17543=CARTESIAN_POINT('Ctrl Pts',(-6.00574667762962,0.353081681743826,
-1.68804235373829));
#17544=CARTESIAN_POINT('Ctrl Pts',(-5.92707607206732,1.60409711297163,-0.633266219818969));
#17545=CARTESIAN_POINT('Ctrl Pts',(-5.84840546650504,1.41096453880922,0.991631343348807));
#17546=CARTESIAN_POINT('Ctrl Pts',(-5.76973486094274,-0.0524412649270098,
1.72377596233671));
#17547=CARTESIAN_POINT('Ctrl Pts',(-5.69106425538045,-1.46863487270643,
0.90402724721636));
#17548=CARTESIAN_POINT('Ctrl Pts',(-5.61239364981816,-1.56263538965757,
-0.729605572830212));
#17549=CARTESIAN_POINT('Ctrl Pts',(-5.53372304425587,-0.249815359540411,
-1.70638387813377));
#17550=CARTESIAN_POINT('Ctrl Pts',(-5.45505243869358,1.28791022644179,-1.1469267203217));
#17551=CARTESIAN_POINT('Ctrl Pts',(-5.37638183313129,1.66614679689841,0.445093815229617));
#17552=CARTESIAN_POINT('Ctrl Pts',(-5.297711227569,0.544372831292141,1.63640211249766));
#17553=CARTESIAN_POINT('Ctrl Pts',(-5.21904062200671,-1.06749299418725,
1.35447863052787));
#17554=CARTESIAN_POINT('Ctrl Pts',(-5.14037001644442,-1.71830860400367,
-0.14686454510099));
#17555=CARTESIAN_POINT('Ctrl Pts',(-5.06169941088213,-0.822153073557281,
-1.51598745933111));
#17556=CARTESIAN_POINT('Ctrl Pts',(-4.98302880531984,0.814176296857773,
-1.52028635816996));
#17557=CARTESIAN_POINT('Ctrl Pts',(-4.90435819975755,1.71751321679322,-0.155890998279683));
#17558=CARTESIAN_POINT('Ctrl Pts',(-4.82568759419526,1.07459507334092,1.34885102274358));
#17559=CARTESIAN_POINT('Ctrl Pts',(-4.74701698863297,-0.535767196304556,
1.63923981301333));
#17560=CARTESIAN_POINT('Ctrl Pts',(-4.66834638307067,-1.66378514860608,
0.453842078792031));
#17561=CARTESIAN_POINT('Ctrl Pts',(-4.58967577750839,-1.29391872641317,
-1.14014384296093));
#17562=CARTESIAN_POINT('Ctrl Pts',(-4.51100517194609,0.240846086526641,
-1.70767292413062));
#17563=CARTESIAN_POINT('Ctrl Pts',(-4.43233456638381,1.55878026483299,-0.737806030859172));
#17564=CARTESIAN_POINT('Ctrl Pts',(-4.35366396082151,1.47336461523605,0.896298144466647));
#17565=CARTESIAN_POINT('Ctrl Pts',(-4.27499335525922,0.0614977487001475,
1.72347662592433));
#17566=CARTESIAN_POINT('Ctrl Pts',(-4.19632274969694,-1.40573475018597,
0.999031263438967));
#17567=CARTESIAN_POINT('Ctrl Pts',(-4.11765214413464,-1.60740232997359,
-0.624829098871234));
#17568=CARTESIAN_POINT('Ctrl Pts',(-4.03898153857236,-0.361946261855135,
-1.68616385820732));
#17569=CARTESIAN_POINT('Ctrl Pts',(-3.96031093301006,1.20936537151692,-1.22946697857712));
#17570=CARTESIAN_POINT('Ctrl Pts',(-3.88164032744778,1.69190091225119,0.334103212037918));
#17571=CARTESIAN_POINT('Ctrl Pts',(-3.80296972188548,0.651239818068822,
1.59688457708217));
#17572=CARTESIAN_POINT('Ctrl Pts',(-3.72429911632319,-0.975724110039982,
1.4220112919748));
#17573=CARTESIAN_POINT('Ctrl Pts',(-3.6456285107609,-1.72425616866463,-0.0330804736536309));
#17574=CARTESIAN_POINT('Ctrl Pts',(-3.56695790519861,-0.920462571341124,
-1.45839031394175));
#17575=CARTESIAN_POINT('Ctrl Pts',(-3.48828729963632,0.712011643205295,
-1.57073010875106));
#17576=CARTESIAN_POINT('Ctrl Pts',(-3.40961669407403,1.70347093011839,-0.26896178377321));
#17577=CARTESIAN_POINT('Ctrl Pts',(-3.33094608851174,1.16131724584182,1.27494937449222));
#17578=CARTESIAN_POINT('Ctrl Pts',(-3.25227548294945,-0.426355425311021,
1.67104000948667));
#17579=CARTESIAN_POINT('Ctrl Pts',(-3.17360487738716,-1.63018578209101,
0.562714804662844));
#17580=CARTESIAN_POINT('Ctrl Pts',(-3.09493427182487,-1.36638085629297,
-1.05221528877668));
#17581=CARTESIAN_POINT('Ctrl Pts',(-3.01626366626258,0.12755921119296,-1.71984951493929));
#17582=CARTESIAN_POINT('Ctrl Pts',(-2.93759306070029,1.50665930937299,-0.839125287818249));
#17583=CARTESIAN_POINT('Ctrl Pts',(-2.858922455138,1.52933350411271,0.797052549027277));
#17584=CARTESIAN_POINT('Ctrl Pts',(-2.78025184957571,0.175168223579021,
1.71565440895862));
#17585=CARTESIAN_POINT('Ctrl Pts',(-2.70158124401342,-1.33669839961298,
1.08967431699807));
#17586=CARTESIAN_POINT('Ctrl Pts',(-2.62291063845113,-1.64515332070094,
-0.517324885749805));
#17587=CARTESIAN_POINT('Ctrl Pts',(-2.54424003288884,-0.472496571810804,
-1.65858441058862));
#17588=CARTESIAN_POINT('Ctrl Pts',(-2.46556942732655,1.12554030939224,-1.30663931286933));
#17589=CARTESIAN_POINT('Ctrl Pts',(-2.38689882176426,1.71027239512204,0.221651779091063));
#17590=CARTESIAN_POINT('Ctrl Pts',(-2.30822821620197,0.755259347912122,
1.55040133257893));
#17591=CARTESIAN_POINT('Ctrl Pts',(-2.22955761063968,-0.879687067669174,
1.48332793536745));
#17592=CARTESIAN_POINT('Ctrl Pts',(-2.15088700507738,-1.72269470217952,
0.0808649939243594));
#17593=CARTESIAN_POINT('Ctrl Pts',(-2.0722163995151,-1.01472123450027,-1.39445963496725));
#17594=CARTESIAN_POINT('Ctrl Pts',(-1.9935457939528,0.606676244407784,-1.6142560781525));
#17595=CARTESIAN_POINT('Ctrl Pts',(-1.91487518839052,1.68211251252115,-0.380975660890149));
#17596=CARTESIAN_POINT('Ctrl Pts',(-1.83620458282822,1.24274270731752,1.19570559574748));
#17597=CARTESIAN_POINT('Ctrl Pts',(-1.75753397726594,-0.314648347061551,
1.6951199455559));
#17598=CARTESIAN_POINT('Ctrl Pts',(-1.67886337170364,-1.5903081925567,0.669957906677155));
#17599=CARTESIAN_POINT('Ctrl Pts',(-1.60019276614136,-1.43118788486783,
-0.96140157819741));
#17600=CARTESIAN_POINT('Ctrl Pts',(-1.54774569576649,-0.470619529268327,
-1.46728923472753));
#17601=CARTESIAN_POINT('Ctrl Pts',(-1.52152216057906,0.0116391963891266,
-1.46345371607968));
#17602=CARTESIAN_POINT('Ctrl Pts',(-2.14715504584291,-1.46566693596749,
0.000405098676182412));
#17603=CARTESIAN_POINT('Ctrl Pts',(-2.12217549706697,-1.46397116480163,
-0.45709640867042));
#17604=CARTESIAN_POINT('Ctrl Pts',(-2.09719594829103,-1.23229569088932,
-0.91608689002793));
#17605=CARTESIAN_POINT('Ctrl Pts',(-2.0722163995151,-0.862483899295466,
-1.18520493734953));
#17606=CARTESIAN_POINT('Ctrl Pts',(-2.04599286432767,-0.474255408197588,
-1.467725116029));
#17607=CARTESIAN_POINT('Ctrl Pts',(-2.01976932914024,0.0662104181050797,
-1.54099059709075));
#17608=CARTESIAN_POINT('Ctrl Pts',(-1.99354579395281,0.51568270927531,-1.37207660141124));
#17609=CARTESIAN_POINT('Ctrl Pts',(-1.96732225876538,0.965155000445553,
-1.20316260573173));
#17610=CARTESIAN_POINT('Ctrl Pts',(-1.94109872357795,1.32363375648335,-0.792069133310953));
#17611=CARTESIAN_POINT('Ctrl Pts',(-1.91487518839052,1.42964483363498,-0.323742187660957));
#17612=CARTESIAN_POINT('Ctrl Pts',(-1.88865165320309,1.53565591078661,0.14458475798904));
#17613=CARTESIAN_POINT('Ctrl Pts',(-1.86242811801566,1.38919930905206,0.670145176868271));
#17614=CARTESIAN_POINT('Ctrl Pts',(-1.83620458282822,1.05640583245494,1.01616111127595));
#17615=CARTESIAN_POINT('Ctrl Pts',(-1.8099810476408,0.723612355857827,1.36217704568362));
#17616=CARTESIAN_POINT('Ctrl Pts',(-1.78375751245337,0.204482004398144,
1.52864849561976));
#17617=CARTESIAN_POINT('Ctrl Pts',(-1.75753397726594,-0.267693145580892,
1.44102388077471));
#17618=CARTESIAN_POINT('Ctrl Pts',(-1.73385598484396,-0.694033817925085,
1.3619050681718));
#17619=CARTESIAN_POINT('Ctrl Pts',(-1.71017799242198,-1.0820928104985,1.07562658259897));
#17620=CARTESIAN_POINT('Ctrl Pts',(-1.6865,-1.29040238558681,0.694864466152488));
#17621=CARTESIAN_POINT('',(-7.7365,-0.684664424539443,-0.95829519891841));
#17622=CARTESIAN_POINT('Ctrl Pts',(-7.7365,-0.686089228034751,-0.959351223124451));
#17623=CARTESIAN_POINT('Ctrl Pts',(-7.7365,-0.719567521781266,-0.941182198525624));
#17624=CARTESIAN_POINT('Ctrl Pts',(-7.7365,-0.752028806414924,-0.921351335407023));
#17625=CARTESIAN_POINT('Ctrl Pts',(-7.7365,-0.783331577414887,-0.899889939916658));
#17626=CARTESIAN_POINT('Ctrl Pts',(-7.7365,-0.823255286032892,-0.872517970192505));
#17627=CARTESIAN_POINT('Ctrl Pts',(-7.7365,-0.861295942401313,-0.842495516275831));
#17628=CARTESIAN_POINT('Ctrl Pts',(-7.7365,-0.897382909658782,-0.810117125580153));
#17629=CARTESIAN_POINT('Ctrl Pts',(-7.7365,-0.910704143482914,-0.798164885032232));
#17630=CARTESIAN_POINT('Ctrl Pts',(-7.7365,-0.923758957569899,-0.785891136787456));
#17631=CARTESIAN_POINT('Ctrl Pts',(-7.7365,-0.93654302005363,-0.773309146568843));
#17632=CARTESIAN_POINT('Ctrl Pts',(-7.7365,-0.944204342863284,-0.765768923046361));
#17633=CARTESIAN_POINT('Ctrl Pts',(-7.7365,-0.951765482935571,-0.75812076753032));
#17634=CARTESIAN_POINT('Ctrl Pts',(-7.7365,-0.959220174508566,-0.750373653173739));
#17635=CARTESIAN_POINT('Ctrl Pts',(-7.7365,-0.994284459823726,-0.713933912440213));
#17636=CARTESIAN_POINT('Ctrl Pts',(-7.7365,-1.02703314687708,-0.675271898636465));
#17637=CARTESIAN_POINT('Ctrl Pts',(-7.7365,-1.05739069023667,-0.634712603653476));
#17638=CARTESIAN_POINT('Ctrl Pts',(-7.7365,-1.07909989922968,-0.605707944054868));
#17639=CARTESIAN_POINT('Ctrl Pts',(-7.7365,-1.09958591366534,-0.575731842990991));
#17640=CARTESIAN_POINT('Ctrl Pts',(-7.7365,-1.11881249318271,-0.54488942520468));
#17641=CARTESIAN_POINT('Ctrl Pts',(-7.7365,-1.12494218476806,-0.535056448485871));
#17642=CARTESIAN_POINT('Ctrl Pts',(-7.7365,-1.13094380182462,-0.525135342523029));
#17643=CARTESIAN_POINT('Ctrl Pts',(-7.7365,-1.13681598362796,-0.515129316344604));
#17644=CARTESIAN_POINT('Ctrl Pts',(-7.7365,-1.14155088186925,-0.507061188118799));
#17645=CARTESIAN_POINT('Ctrl Pts',(-7.7365,-1.14620080441806,-0.498939107641481));
#17646=CARTESIAN_POINT('Ctrl Pts',(-7.7365,-1.15076055599585,-0.490773281325137));
#17647=CARTESIAN_POINT('Ctrl Pts',(-7.7365,-1.17633138736302,-0.444979784871117));
#17648=CARTESIAN_POINT('Ctrl Pts',(-7.7365,-1.19911090769331,-0.397742968678235));
#17649=CARTESIAN_POINT('Ctrl Pts',(-7.7365,-1.2190202952071,-0.349393168832874));
#17650=CARTESIAN_POINT('Ctrl Pts',(-7.7365,-1.2393257464617,-0.30008153113184));
#17651=CARTESIAN_POINT('Ctrl Pts',(-7.7365,-1.25664650233717,-0.249611304674763));
#17652=CARTESIAN_POINT('Ctrl Pts',(-7.7365,-1.27086282858701,-0.198293772224332));
#17653=CARTESIAN_POINT('Ctrl Pts',(-7.7365,-1.27935267763108,-0.167647450793473));
#17654=CARTESIAN_POINT('Ctrl Pts',(-7.7365,-1.2867346336525,-0.136698263002545));
#17655=CARTESIAN_POINT('Ctrl Pts',(-7.7365,-1.29297548212098,-0.105508124729707));
#17656=CARTESIAN_POINT('Ctrl Pts',(-7.7365,-1.29611179238721,-0.0898336613351524));
#17657=CARTESIAN_POINT('Ctrl Pts',(-7.7365,-1.29895981553652,-0.0740983053561009));
#17658=CARTESIAN_POINT('Ctrl Pts',(-7.7365,-1.30151470570495,-0.0583097264166406));
#17659=CARTESIAN_POINT('Ctrl Pts',(-7.7365,-1.30342781450681,-0.0464871949783093));
#17660=CARTESIAN_POINT('Ctrl Pts',(-7.7365,-1.30517672269469,-0.0346323680336482));
#17661=CARTESIAN_POINT('Ctrl Pts',(-7.7365,-1.3067565281468,-0.0227722525703492));
#17662=CARTESIAN_POINT('Ctrl Pts',(-7.7365,-1.31399492195315,0.0315687336550901));
#17663=CARTESIAN_POINT('Ctrl Pts',(-7.7365,-1.31770532384574,0.086122873391717));
#17664=CARTESIAN_POINT('Ctrl Pts',(-7.7365,-1.31777798642413,0.140559222914643));
#17665=CARTESIAN_POINT('Ctrl Pts',(-7.7365,-1.31779471615732,0.153092573965366));
#17666=CARTESIAN_POINT('Ctrl Pts',(-7.7365,-1.31761842432871,0.165619795498501));
#17667=CARTESIAN_POINT('Ctrl Pts',(-7.7365,-1.31724742365147,0.178137029012559));
#17668=CARTESIAN_POINT('Ctrl Pts',(-7.7365,-1.31568993550475,0.230685296506085));
#17669=CARTESIAN_POINT('Ctrl Pts',(-7.7365,-1.31070510000365,0.283056976251484));
#17670=CARTESIAN_POINT('Ctrl Pts',(-7.7365,-1.3024938347724,0.335034845453329));
#17671=CARTESIAN_POINT('Ctrl Pts',(-7.7365,-1.29853419969743,0.360099605659894));
#17672=CARTESIAN_POINT('Ctrl Pts',(-7.7365,-1.293823524476,0.385072900683143));
#17673=CARTESIAN_POINT('Ctrl Pts',(-7.7365,-1.28838015099446,0.409930549200139));
#17674=CARTESIAN_POINT('Ctrl Pts',(-7.7365,-1.28491491105284,0.425754875197221));
#17675=CARTESIAN_POINT('Ctrl Pts',(-7.7365,-1.28115268656436,0.441532333910416));
#17676=CARTESIAN_POINT('Ctrl Pts',(-7.7365,-1.27709766589713,0.457256627308522));
#17677=CARTESIAN_POINT('Ctrl Pts',(-7.7365,-1.27467681968889,0.466644026084986));
#17678=CARTESIAN_POINT('Ctrl Pts',(-7.7365,-1.27215179327647,0.476011400153136));
#17679=CARTESIAN_POINT('Ctrl Pts',(-7.7365,-1.26952717248285,0.485345283174778));
#17680=CARTESIAN_POINT('Ctrl Pts',(-7.7365,-1.25469068744454,0.538107958886544));
#17681=CARTESIAN_POINT('Ctrl Pts',(-7.7365,-1.23664997241023,0.589903525989738));
#17682=CARTESIAN_POINT('Ctrl Pts',(-7.7365,-1.21564557967939,0.640497721438812));
#17683=CARTESIAN_POINT('Ctrl Pts',(-7.7365,-1.19418321507496,0.692195053683102));
#17684=CARTESIAN_POINT('Ctrl Pts',(-7.7365,-1.16962630514638,0.742639006673555));
#17685=CARTESIAN_POINT('Ctrl Pts',(-7.7365,-1.14217654454016,0.791579858150175));
#17686=CARTESIAN_POINT('Ctrl Pts',(-7.7365,-1.12677101513637,0.819046754393308));
#17687=CARTESIAN_POINT('Ctrl Pts',(-7.7365,-1.11045334684977,0.846040134726086));
#17688=CARTESIAN_POINT('Ctrl Pts',(-7.7365,-1.09325230130699,0.872514108250645));
#17689=CARTESIAN_POINT('Ctrl Pts',(-7.7365,-1.08168342987847,0.890319653567393));
#17690=CARTESIAN_POINT('Ctrl Pts',(-7.7365,-1.06971486463694,0.907890215817321));
#17691=CARTESIAN_POINT('Ctrl Pts',(-7.7365,-1.05735420050082,0.925211267082703));
#17692=CARTESIAN_POINT('Ctrl Pts',(-7.7365,-1.04835406887479,0.937823189838047));
#17693=CARTESIAN_POINT('Ctrl Pts',(-7.7365,-1.03914164703506,0.950308284381235));
#17694=CARTESIAN_POINT('Ctrl Pts',(-7.7365,-1.02974297658215,0.962630950059377));
#17695=CARTESIAN_POINT('Ctrl Pts',(-7.7365,-0.994436227831979,1.00892188697543));
#17696=CARTESIAN_POINT('Ctrl Pts',(-7.7365,-0.95646308818278,1.0529859052567));
#17697=CARTESIAN_POINT('Ctrl Pts',(-7.7365,-0.916048129859651,1.09456438762751));
#17698=CARTESIAN_POINT('Ctrl Pts',(-7.7365,-0.874058720315396,1.13776264878959));
#17699=CARTESIAN_POINT('Ctrl Pts',(-7.7365,-0.829433298073862,1.17827929017471));
#17700=CARTESIAN_POINT('Ctrl Pts',(-7.7365,-0.782368886781381,1.21580225379033));
#17701=CARTESIAN_POINT('Ctrl Pts',(-7.7365,-0.738128427827426,1.2510737696997));
#17702=CARTESIAN_POINT('Ctrl Pts',(-7.7365,-0.691731985554792,1.28370079840323));
#17703=CARTESIAN_POINT('Ctrl Pts',(-7.7365,-0.643305397356536,1.31339079617938));
#17704=CARTESIAN_POINT('Ctrl Pts',(-7.7365,-0.640214236454891,1.31528596500523));
#17705=CARTESIAN_POINT('Ctrl Pts',(-7.7365,-0.637114792741105,1.31716915284921));
#17706=CARTESIAN_POINT('Ctrl Pts',(-7.7365,-0.634007094575211,1.31904027763685));
#17707=CARTESIAN_POINT('Ctrl Pts',(-7.7365,-0.686089228034766,-0.959351223124441));
#17708=CARTESIAN_POINT('Ctrl Pts',(-7.71282200757802,-0.400645460942403,
-1.16063686443021));
#17709=CARTESIAN_POINT('Ctrl Pts',(-7.66292047996862,0.404068774457181,
-1.30672719507535));
#17710=CARTESIAN_POINT('Ctrl Pts',(-7.58679541717176,1.32164391460705,-0.423509280609249));
#17711=CARTESIAN_POINT('Ctrl Pts',(-7.50812481160949,1.08034427095369,0.871377146278108));
#17712=CARTESIAN_POINT('Ctrl Pts',(-7.42945420604718,-0.133733706588163,
1.38132579741601));
#17713=CARTESIAN_POINT('Ctrl Pts',(-7.36412356393198,-1.0418916265847,0.772281661640888));
#17714=CARTESIAN_POINT('Ctrl Pts',(-7.32501645700419,-1.1759714297419,0.191448115784734));
#17715=CARTESIAN_POINT('Ctrl Pts',(-7.31213288526384,-1.17589382943587,
6.05154992187017E-5));
#17716=CARTESIAN_POINT('Origin',(-7.7365,-3.28582941601228E-17,0.));
#17717=CARTESIAN_POINT('',(-7.7365,-1.4635,-1.79227059055215E-16));
#17718=CARTESIAN_POINT('Origin',(-7.7365,0.,0.));
#17719=CARTESIAN_POINT('Origin',(-7.7365,0.,0.));
#17720=CARTESIAN_POINT('',(-7.7365,0.684664424539464,-0.958295198918394));
#17721=CARTESIAN_POINT('Ctrl Pts',(-7.7365,0.635526523537867,1.32063649424652));
#17722=CARTESIAN_POINT('Ctrl Pts',(-7.7365,0.675662324545726,1.29678049687132));
#17723=CARTESIAN_POINT('Ctrl Pts',(-7.7365,0.714498513993556,1.27094851430042));
#17724=CARTESIAN_POINT('Ctrl Pts',(-7.7365,0.751863241629522,1.24313459901083));
#17725=CARTESIAN_POINT('Ctrl Pts',(-7.7365,0.79761838124666,1.20907494816116));
#17726=CARTESIAN_POINT('Ctrl Pts',(-7.7365,0.841168365500316,1.172043366427));
#17727=CARTESIAN_POINT('Ctrl Pts',(-7.7365,0.882365785843323,1.1323407093949));
#17728=CARTESIAN_POINT('Ctrl Pts',(-7.7365,0.894337253798062,1.12080360142988));
#17729=CARTESIAN_POINT('Ctrl Pts',(-7.7365,0.906109798442489,1.10904078506667));
#17730=CARTESIAN_POINT('Ctrl Pts',(-7.7365,0.917679117349396,1.09705931043964));
#17731=CARTESIAN_POINT('Ctrl Pts',(-7.7365,0.929420235508159,1.08489991623119));
#17732=CARTESIAN_POINT('Ctrl Pts',(-7.7365,0.940955256724849,1.07251147301931));
#17733=CARTESIAN_POINT('Ctrl Pts',(-7.7365,0.952259483692321,1.05992418359167));
#17734=CARTESIAN_POINT('Ctrl Pts',(-7.7365,0.990695550087743,1.01712551247765));
#17735=CARTESIAN_POINT('Ctrl Pts',(-7.7365,1.0265099806289,0.97198836055672));
#17736=CARTESIAN_POINT('Ctrl Pts',(-7.7365,1.05955705108154,0.924827743938838));
#17737=CARTESIAN_POINT('Ctrl Pts',(-7.7365,1.08185203767515,0.893011147162164));
#17738=CARTESIAN_POINT('Ctrl Pts',(-7.7365,1.10288656680039,0.860272923873848));
#17739=CARTESIAN_POINT('Ctrl Pts',(-7.7365,1.12260321028108,0.826705490119863));
#17740=CARTESIAN_POINT('Ctrl Pts',(-7.7365,1.13151746735871,0.811529036064046));
#17741=CARTESIAN_POINT('Ctrl Pts',(-7.7365,1.14016218873329,0.796183054892689));
#17742=CARTESIAN_POINT('Ctrl Pts',(-7.7365,1.14853132555903,0.780676014340111));
#17743=CARTESIAN_POINT('Ctrl Pts',(-7.7365,1.15371651111356,0.77106846647216));
#17744=CARTESIAN_POINT('Ctrl Pts',(-7.7365,1.15879588965814,0.761398888166361));
#17745=CARTESIAN_POINT('Ctrl Pts',(-7.7365,1.1637615407048,0.751682494664184));
#17746=CARTESIAN_POINT('Ctrl Pts',(-7.7365,1.18936063251987,0.701592215054026));
#17747=CARTESIAN_POINT('Ctrl Pts',(-7.7365,1.21198804521927,0.650173906188369));
#17748=CARTESIAN_POINT('Ctrl Pts',(-7.7365,1.23150471893565,0.597718969633297));
#17749=CARTESIAN_POINT('Ctrl Pts',(-7.7365,1.2505456032793,0.546542811507523));
#17750=CARTESIAN_POINT('Ctrl Pts',(-7.7365,1.26662568914227,0.494378903403244));
#17751=CARTESIAN_POINT('Ctrl Pts',(-7.7365,1.27956755855888,0.441492195363456));
#17752=CARTESIAN_POINT('Ctrl Pts',(-7.7365,1.28740987234878,0.409444726299148));
#17753=CARTESIAN_POINT('Ctrl Pts',(-7.7365,1.29409891046221,0.377131810910926));
#17754=CARTESIAN_POINT('Ctrl Pts',(-7.7365,1.29958594646738,0.34461372675715));
#17755=CARTESIAN_POINT('Ctrl Pts',(-7.7365,1.30228746124199,0.328603610420976));
#17756=CARTESIAN_POINT('Ctrl Pts',(-7.7365,1.30469749609525,0.312543786613891));
#17757=CARTESIAN_POINT('Ctrl Pts',(-7.7365,1.30680957950161,0.296441647110286));
#17758=CARTESIAN_POINT('Ctrl Pts',(-7.7365,1.30814831885088,0.286235341954064));
#17759=CARTESIAN_POINT('Ctrl Pts',(-7.7365,1.3093675450585,0.276010135619152));
#17760=CARTESIAN_POINT('Ctrl Pts',(-7.7365,1.31046487898323,0.26577397180974));
#17761=CARTESIAN_POINT('Ctrl Pts',(-7.7365,1.31610218862947,0.213187950651897));
#17762=CARTESIAN_POINT('Ctrl Pts',(-7.7365,1.31850650693356,0.160512130657276));
#17763=CARTESIAN_POINT('Ctrl Pts',(-7.7365,1.31752770333829,0.107993690563324));
#17764=CARTESIAN_POINT('Ctrl Pts',(-7.7365,1.31716603454866,0.0885880807409719));
#17765=CARTESIAN_POINT('Ctrl Pts',(-7.7365,1.31634196331213,0.069204000142364));
#17766=CARTESIAN_POINT('Ctrl Pts',(-7.7365,1.31504611373144,0.049854209528768));
#17767=CARTESIAN_POINT('Ctrl Pts',(-7.7365,1.31152658503734,-0.00269984018871856));
#17768=CARTESIAN_POINT('Ctrl Pts',(-7.7365,1.30452994593076,-0.0550026064406229));
#17769=CARTESIAN_POINT('Ctrl Pts',(-7.7365,1.29420811169353,-0.106785251320807));
#17770=CARTESIAN_POINT('Ctrl Pts',(-7.7365,1.28945298735972,-0.130640789888765));
#17771=CARTESIAN_POINT('Ctrl Pts',(-7.7365,1.28399154727714,-0.154385628993537));
#17772=CARTESIAN_POINT('Ctrl Pts',(-7.7365,1.27783584092355,-0.177991493805362));
#17773=CARTESIAN_POINT('Ctrl Pts',(-7.7365,1.27344015870932,-0.194848028887567));
#17774=CARTESIAN_POINT('Ctrl Pts',(-7.7365,1.26869042478761,-0.211633671496613));
#17775=CARTESIAN_POINT('Ctrl Pts',(-7.7365,1.26359055949064,-0.228337623457783));
#17776=CARTESIAN_POINT('Ctrl Pts',(-7.7365,1.26062482770685,-0.238051495954687));
#17777=CARTESIAN_POINT('Ctrl Pts',(-7.7365,1.25754318746128,-0.247729405397701));
#17778=CARTESIAN_POINT('Ctrl Pts',(-7.7365,1.25434848629719,-0.257365044593482));
#17779=CARTESIAN_POINT('Ctrl Pts',(-7.7365,1.23782735626646,-0.307194947268678));
#17780=CARTESIAN_POINT('Ctrl Pts',(-7.7365,1.21827446902308,-0.355935352114231));
#17781=CARTESIAN_POINT('Ctrl Pts',(-7.7365,1.19586331884282,-0.403328860609973));
#17782=CARTESIAN_POINT('Ctrl Pts',(-7.7365,1.17355664767014,-0.450501424321841));
#17783=CARTESIAN_POINT('Ctrl Pts',(-7.7365,1.14841750560847,-0.496340514203069));
#17784=CARTESIAN_POINT('Ctrl Pts',(-7.7365,1.12057781089321,-0.540559531039698));
#17785=CARTESIAN_POINT('Ctrl Pts',(-7.7365,1.10664317367144,-0.562692530852515));
#17786=CARTESIAN_POINT('Ctrl Pts',(-7.7365,1.09203142308822,-0.584419053510079));
#17787=CARTESIAN_POINT('Ctrl Pts',(-7.7365,1.07675632505549,-0.605698999841668));
#17788=CARTESIAN_POINT('Ctrl Pts',(-7.7365,1.0654995981464,-0.621380898837115));
#17789=CARTESIAN_POINT('Ctrl Pts',(-7.7365,1.05388258904147,-0.636820217291134));
#17790=CARTESIAN_POINT('Ctrl Pts',(-7.7365,1.04191030972442,-0.651999766019219));
#17791=CARTESIAN_POINT('Ctrl Pts',(-7.7365,1.03612119897676,-0.659339729142309));
#17792=CARTESIAN_POINT('Ctrl Pts',(-7.7365,1.03024956724999,-0.666618087250615));
#17793=CARTESIAN_POINT('Ctrl Pts',(-7.7365,1.02430436591076,-0.673823161713142));
#17794=CARTESIAN_POINT('Ctrl Pts',(-7.7365,0.992204746549825,-0.71272514913416));
#17795=CARTESIAN_POINT('Ctrl Pts',(-7.7365,0.957901230445239,-0.74957321341277));
#17796=CARTESIAN_POINT('Ctrl Pts',(-7.7365,0.92152517839075,-0.784115990711642));
#17797=CARTESIAN_POINT('Ctrl Pts',(-7.7365,0.885896112329949,-0.817949428503667));
#17798=CARTESIAN_POINT('Ctrl Pts',(-7.7365,0.848278005670964,-0.849571861278115));
#17799=CARTESIAN_POINT('Ctrl Pts',(-7.7365,0.808770590985111,-0.878703555606754));
#17800=CARTESIAN_POINT('Ctrl Pts',(-7.7365,0.769263176299258,-0.907835249935393));
#17801=CARTESIAN_POINT('Ctrl Pts',(-7.7365,0.727865824984928,-0.934476884924097));
#17802=CARTESIAN_POINT('Ctrl Pts',(-7.7365,0.684664424539481,-0.958295198918382));
#17803=CARTESIAN_POINT('Origin',(-7.7365,0.,0.));
#17804=CARTESIAN_POINT('Origin',(-8.66086711473615,0.,0.));
#17805=CARTESIAN_POINT('Ctrl Pts',(-7.7365,0.684664424539464,-0.958295198918394));
#17806=CARTESIAN_POINT('Ctrl Pts',(-7.71027646481257,1.00045590899587,-0.732674539205356));
#17807=CARTESIAN_POINT('Ctrl Pts',(-7.65782939443771,1.38654401896136,0.0510548484666211));
#17808=CARTESIAN_POINT('Ctrl Pts',(-7.57915878887542,0.718476098825324,
1.1884261498247));
#17809=CARTESIAN_POINT('Ctrl Pts',(-7.50048818331313,-0.596971468671329,
1.25245241149886));
#17810=CARTESIAN_POINT('Ctrl Pts',(-7.44439095860004,-1.15153259873763,
0.495303688165933));
#17811=CARTESIAN_POINT('Ctrl Pts',(-7.41451726907438,-1.17920005900012,
0.0547824536253384));
#17812=CARTESIAN_POINT('Ctrl Pts',(-7.41086711473616,-1.17877062515776,
0.00089983691722877));
#17813=CARTESIAN_POINT('Ctrl Pts',(-7.90147783942094,0.850780204044563,
-1.1908002747757));
#17814=CARTESIAN_POINT('Ctrl Pts',(-7.87525430423351,1.24319017008315,-0.910438707813255));
#17815=CARTESIAN_POINT('Ctrl Pts',(-7.82280723385863,1.72295238526848,0.0634419619875768));
#17816=CARTESIAN_POINT('Ctrl Pts',(-7.74413662829637,0.892795390049576,
1.47676643622877));
#17817=CARTESIAN_POINT('Ctrl Pts',(-7.66546602273406,-0.741810863426415,
1.5563269830003));
#17818=CARTESIAN_POINT('Ctrl Pts',(-7.58679541717177,-1.70821806364401,
0.236880057866908));
#17819=CARTESIAN_POINT('Ctrl Pts',(-7.50812481160949,-1.1369258247315,-1.2969366021893));
#17820=CARTESIAN_POINT('Ctrl Pts',(-7.42945420604719,0.458024564052897,
-1.66255611650173));
#17821=CARTESIAN_POINT('Ctrl Pts',(-7.35078360048491,1.64056958905846,-0.531703329058153));
#17822=CARTESIAN_POINT('Ctrl Pts',(-7.27211299492261,1.3461580990934,1.07799570430111));
#17823=CARTESIAN_POINT('Ctrl Pts',(-7.19344238936033,-0.160196505892506,
1.7171046833336));
#17824=CARTESIAN_POINT('Ctrl Pts',(-7.11477178379802,-1.52232074755266,
0.810370741545469));
#17825=CARTESIAN_POINT('Ctrl Pts',(-7.03610117823575,-1.51392314204059,
-0.82595286244993));
#17826=CARTESIAN_POINT('Ctrl Pts',(-6.95743057267345,-0.142557925666395,
-1.71866947855556));
#17827=CARTESIAN_POINT('Ctrl Pts',(-6.87875996711116,1.35714926820058,-1.06409649964009));
#17828=CARTESIAN_POINT('Ctrl Pts',(-6.80008936154887,1.63503300035843,0.548472256796127));
#17829=CARTESIAN_POINT('Ctrl Pts',(-6.72141875598658,0.440917246385971,
1.66725671587453));
#17830=CARTESIAN_POINT('Ctrl Pts',(-6.64274815042429,-1.15015047653549,
1.28503232716283));
#17831=CARTESIAN_POINT('Ctrl Pts',(-6.564077544862,-1.70575259846417,-0.254090632197126));
#17832=CARTESIAN_POINT('Ctrl Pts',(-6.48540693929971,-0.725687546773451,
-1.56445880480453));
#17833=CARTESIAN_POINT('Ctrl Pts',(-6.40673633373742,0.90770464862602,-1.4663649685594));
#17834=CARTESIAN_POINT('Ctrl Pts',(-6.32806572817513,1.72390203320474,-0.0481215360256416));
#17835=CARTESIAN_POINT('Ctrl Pts',(-6.24939512261284,0.98809257879479,1.41344505915252));
#17836=CARTESIAN_POINT('Ctrl Pts',(-6.17072451705055,-0.637283914981675,
1.6025052628958));
#17837=CARTESIAN_POINT('Ctrl Pts',(-6.09205391148826,-1.68892189675471,
0.348850574905169));
#17838=CARTESIAN_POINT('Ctrl Pts',(-6.01338330592596,-1.22004521199122,
-1.21886979433108));
#17839=CARTESIAN_POINT('Ctrl Pts',(-5.93471270036368,0.347222487949291,
-1.68925736416691));
#17840=CARTESIAN_POINT('Ctrl Pts',(-5.85604209480139,1.6018902472152,-0.63882824988828));
#17841=CARTESIAN_POINT('Ctrl Pts',(-5.77737148923909,1.41439681566205,0.98672972221364));
#17842=CARTESIAN_POINT('Ctrl Pts',(-5.69870088367681,-0.0464598810777479,
1.72394761428674));
#17843=CARTESIAN_POINT('Ctrl Pts',(-5.62003027811451,-1.46548934435283,
0.909117637431074));
#17844=CARTESIAN_POINT('Ctrl Pts',(-5.54135967255222,-1.56515759577583,
-0.724179257845961));
#17845=CARTESIAN_POINT('Ctrl Pts',(-5.46268906698994,-0.255734590265156,
-1.70550687964489));
#17846=CARTESIAN_POINT('Ctrl Pts',(-5.38401846142764,1.28392297834745,-1.15138858896788));
#17847=CARTESIAN_POINT('Ctrl Pts',(-5.30534785586536,1.66768119965738,0.439310042508211));
#17848=CARTESIAN_POINT('Ctrl Pts',(-5.22667725030306,0.550047481812638,
1.63450349185888));
#17849=CARTESIAN_POINT('Ctrl Pts',(-5.14800664474078,-1.06278691078792,
1.35817446574403));
#17850=CARTESIAN_POINT('Ctrl Pts',(-5.06933603917848,-1.71880791409912,
-0.1409015669634));
#17851=CARTESIAN_POINT('Ctrl Pts',(-4.99066543361619,-0.827408254686503,
-1.51312573080365));
#17852=CARTESIAN_POINT('Ctrl Pts',(-4.91199482805391,0.808896416687006,
-1.52310225665036));
#17853=CARTESIAN_POINT('Ctrl Pts',(-4.83332422249161,1.71696204580489,-0.161849406574037));
#17854=CARTESIAN_POINT('Ctrl Pts',(-4.75465361692932,1.07926882368778,1.34511438300187));
#17855=CARTESIAN_POINT('Ctrl Pts',(-4.67598301136703,-0.530076241959179,
1.64108899053431));
#17856=CARTESIAN_POINT('Ctrl Pts',(-4.59731240580474,-1.66220048327908,
0.459612282832222));
#17857=CARTESIAN_POINT('Ctrl Pts',(-4.51864180024245,-1.29786700392053,
-1.13564745289939));
#17858=CARTESIAN_POINT('Ctrl Pts',(-4.43997119468017,0.234919449652514,
-1.70849839020005));
#17859=CARTESIAN_POINT('Ctrl Pts',(-4.36130058911786,1.55621094356038,-0.743210196573115));
#17860=CARTESIAN_POINT('Ctrl Pts',(-4.28262998355559,1.47646573646414,0.891180580009837));
#17861=CARTESIAN_POINT('Ctrl Pts',(-4.20395937799329,0.0674774128713119,
1.7232529401937));
#17862=CARTESIAN_POINT('Ctrl Pts',(-4.125288772431,-1.40225995784398,1.00390283782921));
#17863=CARTESIAN_POINT('Ctrl Pts',(-4.04661816686871,-1.60956072030047,
-0.619248080154418));
#17864=CARTESIAN_POINT('Ctrl Pts',(-3.96794756130641,-0.367794663838479,
-1.68489791451942));
#17865=CARTESIAN_POINT('Ctrl Pts',(-3.88927695574414,1.20509219906104,-1.23365582279537));
#17866=CARTESIAN_POINT('Ctrl Pts',(-3.81060635018183,1.6930500513766,0.328230742601033));
#17867=CARTESIAN_POINT('Ctrl Pts',(-3.73193574461956,0.656776713900384,
1.59461539095066));
#17868=CARTESIAN_POINT('Ctrl Pts',(-3.65326513905725,-0.970784254195621,
1.42538830861477));
#17869=CARTESIAN_POINT('Ctrl Pts',(-3.57459453349497,-1.72436064040639,
-0.0270975396048894));
#17870=CARTESIAN_POINT('Ctrl Pts',(-3.49592392793268,-0.925517318188167,
-1.4551878197274));
#17871=CARTESIAN_POINT('Ctrl Pts',(-3.41725332237038,0.706557348807113,
-1.57319122129186));
#17872=CARTESIAN_POINT('Ctrl Pts',(-3.3385827168081,1.70252751172897,-0.274870790223342));
#17873=CARTESIAN_POINT('Ctrl Pts',(-3.2599121112458,1.16573406527154,1.27091226738214));
#17874=CARTESIAN_POINT('Ctrl Pts',(-3.18124150568352,-0.420554801135517,
1.67250937498041));
#17875=CARTESIAN_POINT('Ctrl Pts',(-3.10257090012123,-1.62822352850371,
0.568367758321523));
#17876=CARTESIAN_POINT('Ctrl Pts',(-3.02390029455893,-1.37002366395617,
-1.04746796454006));
#17877=CARTESIAN_POINT('Ctrl Pts',(-2.94522968899664,0.121591103545963,
-1.72028189668636));
#17878=CARTESIAN_POINT('Ctrl Pts',(-2.86655908343436,1.50373855385807,-0.844347876428985));
#17879=CARTESIAN_POINT('Ctrl Pts',(-2.78788847787206,1.53209030147049,0.791741142594091));
#17880=CARTESIAN_POINT('Ctrl Pts',(-2.70921787230978,0.181119366601109,
1.71503681353074));
#17881=CARTESIAN_POINT('Ctrl Pts',(-2.63054726674748,-1.33290817848094,
1.09430495129436));
#17882=CARTESIAN_POINT('Ctrl Pts',(-2.55187666118519,-1.64694100897837,
-0.511611887997731));
#17883=CARTESIAN_POINT('Ctrl Pts',(-2.47320605562291,-0.478243792685512,
-1.6569381617731));
#17884=CARTESIAN_POINT('Ctrl Pts',(-2.39453545006061,1.12099068518354,-1.31053092209154));
#17885=CARTESIAN_POINT('Ctrl Pts',(-2.31586484449832,1.71104872304431,0.215704968915506));
#17886=CARTESIAN_POINT('Ctrl Pts',(-2.23719423893603,0.760601079226869,
1.54779294640914));
#17887=CARTESIAN_POINT('Ctrl Pts',(-2.15852363337374,-0.874471743967447,
1.48633055233205));
#17888=CARTESIAN_POINT('Ctrl Pts',(-2.07985302781145,-1.72252427571784,
0.0869195064554992));
#17889=CARTESIAN_POINT('Ctrl Pts',(-2.00118242224916,-1.01932419303934,
-1.39107846804535));
#17890=CARTESIAN_POINT('Ctrl Pts',(-1.92251181668687,0.600633420986038,
-1.61606823145153));
#17891=CARTESIAN_POINT('Ctrl Pts',(-1.84384121112458,1.68162810247198,-0.387362415112847));
#17892=CARTESIAN_POINT('Ctrl Pts',(-1.76517060556229,1.24515253395799,1.19255397010835));
#17893=CARTESIAN_POINT('Ctrl Pts',(-1.71272353518743,0.212069491421795,
1.526252590656));
#17894=CARTESIAN_POINT('Ctrl Pts',(-1.6865,-0.26238990830909,1.43978602091337));
#17895=CARTESIAN_POINT('Ctrl Pts',(-7.84648522628062,0.795408277542863,
-1.11329858282327));
#17896=CARTESIAN_POINT('Ctrl Pts',(-7.82026169109319,1.16227874972072,-0.851183984943956));
#17897=CARTESIAN_POINT('Ctrl Pts',(-7.76781462071834,1.61081626316611,0.059312924147259));
#17898=CARTESIAN_POINT('Ctrl Pts',(-7.68914401515604,0.834688959641492,
1.38065300742741));
#17899=CARTESIAN_POINT('Ctrl Pts',(-7.61047340959375,-0.69353106517472,
1.45503545916649));
#17900=CARTESIAN_POINT('Ctrl Pts',(-7.53180280403146,-1.59704090576079,
0.221463026427322));
#17901=CARTESIAN_POINT('Ctrl Pts',(-7.45313219846917,-1.0629304815093,-1.21252716497815));
#17902=CARTESIAN_POINT('Ctrl Pts',(-7.37446159290688,0.42821462915298,-1.5543508072453));
#17903=CARTESIAN_POINT('Ctrl Pts',(-7.2957909873446,1.53379524443405,-0.497098107266011));
#17904=CARTESIAN_POINT('Ctrl Pts',(-7.2171203817823,1.25854514457433,1.00783575156133));
#17905=CARTESIAN_POINT('Ctrl Pts',(-7.13844977622001,-0.149770324009179,
1.60534915132983));
#17906=CARTESIAN_POINT('Ctrl Pts',(-7.05977917065772,-1.4232424754622,0.75762881251765));
#17907=CARTESIAN_POINT('Ctrl Pts',(-6.98110856509543,-1.41539141721697,
-0.772196791286046));
#17908=CARTESIAN_POINT('Ctrl Pts',(-6.90243795953315,-0.133279727907777,
-1.60681210388359));
#17909=CARTESIAN_POINT('Ctrl Pts',(-6.82376735397085,1.26882096769077,-0.994841158614657));
#17910=CARTESIAN_POINT('Ctrl Pts',(-6.74509674840856,1.52861899743111,0.512775651083916));
#17911=CARTESIAN_POINT('Ctrl Pts',(-6.66642614284627,0.41222071907591,1.55874547420248));
#17912=CARTESIAN_POINT('Ctrl Pts',(-6.58775553728398,-1.07529442399706,
1.20139766425729));
#17913=CARTESIAN_POINT('Ctrl Pts',(-6.50908493172169,-1.59473590218558,
-0.237553472841633));
#17914=CARTESIAN_POINT('Ctrl Pts',(-6.4304143261594,-0.678457113681425,
-1.4626380318919));
#17915=CARTESIAN_POINT('Ctrl Pts',(-6.35174372059711,0.84862786845409,-1.37092850579528));
#17916=CARTESIAN_POINT('Ctrl Pts',(-6.27307311503482,1.6117041044977,-0.0449896082453522));
#17917=CARTESIAN_POINT('Ctrl Pts',(-6.19440250947253,0.923783854414734,
1.32145282007889));
#17918=CARTESIAN_POINT('Ctrl Pts',(-6.11573190391023,-0.595807117645157,
1.49820828558741));
#17919=CARTESIAN_POINT('Ctrl Pts',(-6.03706129834795,-1.57900060487505,
0.326146087539453));
#17920=CARTESIAN_POINT('Ctrl Pts',(-5.95839069278565,-1.14064015121761,
-1.13954123409191));
#17921=CARTESIAN_POINT('Ctrl Pts',(-5.87972008722336,0.324623962512216,
-1.57931423882567));
#17922=CARTESIAN_POINT('Ctrl Pts',(-5.80104948166108,1.49763329740499,-0.59725094151666));
#17923=CARTESIAN_POINT('Ctrl Pts',(-5.72237887609879,1.32234263274998,0.922509697587169));
#17924=CARTESIAN_POINT('Ctrl Pts',(-5.64370827053649,-0.0434360999553401,
1.61174671899407));
#17925=CARTESIAN_POINT('Ctrl Pts',(-5.5650376649742,-1.37010987045491,0.849948894714764));
#17926=CARTESIAN_POINT('Ctrl Pts',(-5.48636705941192,-1.46329134295885,
-0.677046989783222));
#17927=CARTESIAN_POINT('Ctrl Pts',(-5.40769645384962,-0.239090436030262,
-1.59450617565708));
#17928=CARTESIAN_POINT('Ctrl Pts',(-5.32902584828734,1.20036051597124,-1.07645195548704));
#17929=CARTESIAN_POINT('Ctrl Pts',(-5.25035524272504,1.55914233100869,0.410718117978727));
#17930=CARTESIAN_POINT('Ctrl Pts',(-5.17168463716275,0.51424835462257,1.52812395130572));
#17931=CARTESIAN_POINT('Ctrl Pts',(-5.09301403160046,-0.993616802654991,
1.26977944158132));
#17932=CARTESIAN_POINT('Ctrl Pts',(-5.01434342603817,-1.6069415295293,-0.131731171163432));
#17933=CARTESIAN_POINT('Ctrl Pts',(-4.93567282047588,-0.773557461205876,
-1.41464590445651));
#17934=CARTESIAN_POINT('Ctrl Pts',(-4.85700221491359,0.756250442181078,
-1.42397312105354));
#17935=CARTESIAN_POINT('Ctrl Pts',(-4.7783316093513,1.60521579717974,-0.151315647792904));
#17936=CARTESIAN_POINT('Ctrl Pts',(-4.69966100378901,1.00902601162336,1.2575693573914));
#17937=CARTESIAN_POINT('Ctrl Pts',(-4.62099039822673,-0.495576917021291,
1.53428084133828));
#17938=CARTESIAN_POINT('Ctrl Pts',(-4.54231979266443,-1.55401831994985,
0.429699013314095));
#17939=CARTESIAN_POINT('Ctrl Pts',(-4.46364918710214,-1.213397012719,-1.06173531085042));
#17940=CARTESIAN_POINT('Ctrl Pts',(-4.38497858153985,0.219630021856553,
-1.59730298762639));
#17941=CARTESIAN_POINT('Ctrl Pts',(-4.30630797597756,1.45492697200307,-0.694839324537859));
#17942=CARTESIAN_POINT('Ctrl Pts',(-4.22763737041527,1.38037187831708,0.833179247419522));
#17943=CARTESIAN_POINT('Ctrl Pts',(-4.14896676485298,0.0630857329423726,
1.6110972568637));
#17944=CARTESIAN_POINT('Ctrl Pts',(-4.07029615929069,-1.31099568658697,
0.938565123238685));
#17945=CARTESIAN_POINT('Ctrl Pts',(-3.9916255537284,-1.50480454769464,-0.578945121743281));
#17946=CARTESIAN_POINT('Ctrl Pts',(-3.91295494816611,-0.343857225006483,
-1.57523851830625));
#17947=CARTESIAN_POINT('Ctrl Pts',(-3.83428434260382,1.12666033574668,-1.15336493306441));
#17948=CARTESIAN_POINT('Ctrl Pts',(-3.75561373704152,1.58286008390573,0.306868270286214));
#17949=CARTESIAN_POINT('Ctrl Pts',(-3.67694313147924,0.614031253019605,
1.49083191572821));
#17950=CARTESIAN_POINT('Ctrl Pts',(-3.59827252591694,-0.907602019681017,
1.33261875863488));
#17951=CARTESIAN_POINT('Ctrl Pts',(-3.51960192035466,-1.61213286384424,
-0.02533393137301));
#17952=CARTESIAN_POINT('Ctrl Pts',(-3.44093131479236,-0.86528122351278,
-1.36047880720329));
#17953=CARTESIAN_POINT('Ctrl Pts',(-3.36226070923008,0.660571979846494,
-1.47080211037416));
#17954=CARTESIAN_POINT('Ctrl Pts',(-3.28359010366778,1.59172071603906,-0.256981181225197));
#17955=CARTESIAN_POINT('Ctrl Pts',(-3.20491949810549,1.0898637750651,1.18819659026007));
#17956=CARTESIAN_POINT('Ctrl Pts',(-3.12624889254321,-0.393183537173681,
1.56365627080078));
#17957=CARTESIAN_POINT('Ctrl Pts',(-3.04757828698091,-1.52225271122323,
0.531376279688018));
#17958=CARTESIAN_POINT('Ctrl Pts',(-2.96890768141862,-1.28085745009089,
-0.979294870161908));
#17959=CARTESIAN_POINT('Ctrl Pts',(-2.89023707585633,0.113677504220552,
-1.60831957987093));
#17960=CARTESIAN_POINT('Ctrl Pts',(-2.81156647029404,1.40586967975149,-0.789394589630305));
#17961=CARTESIAN_POINT('Ctrl Pts',(-2.73289586473175,1.43237619062999,0.74021169685984));
#17962=CARTESIAN_POINT('Ctrl Pts',(-2.65422525916947,0.169331447456067,
1.60341586615199));
#17963=CARTESIAN_POINT('Ctrl Pts',(-2.57555465360717,-1.24615757786577,
1.02308353235976));
#17964=CARTESIAN_POINT('Ctrl Pts',(-2.49688404804488,-1.53975198874934,
-0.478314291597477));
#17965=CARTESIAN_POINT('Ctrl Pts',(-2.41821344248259,-0.447117915505253,
-1.54909848981622));
#17966=CARTESIAN_POINT('Ctrl Pts',(-2.3395428369203,1.04803245985813,-1.22523671619525));
#17967=CARTESIAN_POINT('Ctrl Pts',(-2.26087223135801,1.59968733536411,0.201666090685789));
#17968=CARTESIAN_POINT('Ctrl Pts',(-2.18220162579572,0.71109834414223,1.44705684928207));
#17969=CARTESIAN_POINT('Ctrl Pts',(-2.10353102023343,-0.817557884307119,
1.38959465543445));
#17970=CARTESIAN_POINT('Ctrl Pts',(-2.02486041467114,-1.61041601657051,
0.0812624630732668));
#17971=CARTESIAN_POINT('Ctrl Pts',(-1.94618980910885,-0.95298279953951,
-1.30054192955453));
#17972=CARTESIAN_POINT('Ctrl Pts',(-1.86751920354656,0.561541973532051,
-1.51088852591975));
#17973=CARTESIAN_POINT('Ctrl Pts',(-1.78884859798427,1.57218151773645,-0.362151434559715));
#17974=CARTESIAN_POINT('Ctrl Pts',(-1.71017799242198,1.16411339568706,1.11493814116895));
#17975=CARTESIAN_POINT('Ctrl Pts',(-1.65773092204712,0.198267223531165,
1.42691841965499));
#17976=CARTESIAN_POINT('Ctrl Pts',(-1.63150738685969,-0.245312601328269,
1.34607941449588));
#17977=CARTESIAN_POINT('Ctrl Pts',(-7.79149261314031,0.740036351041164,
-1.03579689087083));
#17978=CARTESIAN_POINT('Ctrl Pts',(-7.76526907795288,1.08136732935829,-0.791929262074656));
#17979=CARTESIAN_POINT('Ctrl Pts',(-7.71282200757803,1.49868014106374,0.0551838863069402));
#17980=CARTESIAN_POINT('Ctrl Pts',(-7.63415140201572,0.776582529233407,
1.28453957862605));
#17981=CARTESIAN_POINT('Ctrl Pts',(-7.55548079645345,-0.645251266923024,
1.35374393533268));
#17982=CARTESIAN_POINT('Ctrl Pts',(-7.47681019089115,-1.48586374787757,
0.206045994987737));
#17983=CARTESIAN_POINT('Ctrl Pts',(-7.39813958532887,-0.98893513828711,
-1.128117727767));
#17984=CARTESIAN_POINT('Ctrl Pts',(-7.31946897976657,0.398404694253064,
-1.44614549798886));
#17985=CARTESIAN_POINT('Ctrl Pts',(-7.24079837420428,1.42702089980965,-0.462492885473871));
#17986=CARTESIAN_POINT('Ctrl Pts',(-7.16212776864199,1.17093219005527,0.937675798821544));
#17987=CARTESIAN_POINT('Ctrl Pts',(-7.0834571630797,-0.13934414212585,1.49359361932605));
#17988=CARTESIAN_POINT('Ctrl Pts',(-7.0047865575174,-1.32416420337174,0.704886883489828));
#17989=CARTESIAN_POINT('Ctrl Pts',(-6.92611595195512,-1.31685969239335,
-0.718440720122158));
#17990=CARTESIAN_POINT('Ctrl Pts',(-6.84744534639283,-0.124001530149162,
-1.49495472921164));
#17991=CARTESIAN_POINT('Ctrl Pts',(-6.76877474083054,1.18049266718097,-0.925585817589218));
#17992=CARTESIAN_POINT('Ctrl Pts',(-6.69010413526825,1.42220499450378,0.477079045371704));
#17993=CARTESIAN_POINT('Ctrl Pts',(-6.61143352970596,0.383524191765849,
1.45023423253043));
#17994=CARTESIAN_POINT('Ctrl Pts',(-6.53276292414367,-1.00043837145862,
1.11776300135174));
#17995=CARTESIAN_POINT('Ctrl Pts',(-6.45409231858137,-1.48371920590699,
-0.221016313486138));
#17996=CARTESIAN_POINT('Ctrl Pts',(-6.37542171301909,-0.631226680589397,
-1.36081725897928));
#17997=CARTESIAN_POINT('Ctrl Pts',(-6.29675110745679,0.789551088282159,
-1.27549204303116));
#17998=CARTESIAN_POINT('Ctrl Pts',(-6.21808050189452,1.49950617579067,-0.0418576804650646));
#17999=CARTESIAN_POINT('Ctrl Pts',(-6.13940989633221,0.859475130034677,
1.22946058100525));
#18000=CARTESIAN_POINT('Ctrl Pts',(-6.06073929076993,-0.554330320308637,
1.39391130827902));
#18001=CARTESIAN_POINT('Ctrl Pts',(-5.98206868520763,-1.46907931299539,
0.303441600173735));
#18002=CARTESIAN_POINT('Ctrl Pts',(-5.90339807964535,-1.06123509044401,
-1.06021267385274));
#18003=CARTESIAN_POINT('Ctrl Pts',(-5.82472747408305,0.302025437075139,
-1.46937111348443));
#18004=CARTESIAN_POINT('Ctrl Pts',(-5.74605686852076,1.39337634759478,-0.555673633145038));
#18005=CARTESIAN_POINT('Ctrl Pts',(-5.66738626295848,1.2302884498379,0.858289672960698));
#18006=CARTESIAN_POINT('Ctrl Pts',(-5.58871565739618,-0.0404123188329307,
1.49954582370141));
#18007=CARTESIAN_POINT('Ctrl Pts',(-5.51004505183389,-1.27473039655699,
0.790780151998455));
#18008=CARTESIAN_POINT('Ctrl Pts',(-5.4313744462716,-1.36142509014187,-0.629914721720484));
#18009=CARTESIAN_POINT('Ctrl Pts',(-5.35270384070931,-0.222446281795369,
-1.48350547166926));
#18010=CARTESIAN_POINT('Ctrl Pts',(-5.27403323514702,1.11679805359503,-1.00151532200621));
#18011=CARTESIAN_POINT('Ctrl Pts',(-5.19536262958473,1.45060346235999,0.382126193449246));
#18012=CARTESIAN_POINT('Ctrl Pts',(-5.11669202402245,0.478449227432503,
1.42174441075256));
#18013=CARTESIAN_POINT('Ctrl Pts',(-5.03802141846014,-0.924446694522063,
1.18138441741861));
#18014=CARTESIAN_POINT('Ctrl Pts',(-4.95935081289786,-1.49507514495947,
-0.122560775363463));
#18015=CARTESIAN_POINT('Ctrl Pts',(-4.88068020733557,-0.719706667725249,
-1.31616607810937));
#18016=CARTESIAN_POINT('Ctrl Pts',(-4.80200960177328,0.703604467675148,
-1.32484398545671));
#18017=CARTESIAN_POINT('Ctrl Pts',(-4.72333899621099,1.49346954855458,-0.140781889011772));
#18018=CARTESIAN_POINT('Ctrl Pts',(-4.6446683906487,0.938783199558951,1.17002433178093));
#18019=CARTESIAN_POINT('Ctrl Pts',(-4.56599778508641,-0.461077592083401,
1.42747269214224));
#18020=CARTESIAN_POINT('Ctrl Pts',(-4.48732717952412,-1.44583615662062,
0.399785743795968));
#18021=CARTESIAN_POINT('Ctrl Pts',(-4.40865657396183,-1.12892702151747,
-0.98782316880146));
#18022=CARTESIAN_POINT('Ctrl Pts',(-4.32998596839954,0.204340594060589,
-1.48610758505272));
#18023=CARTESIAN_POINT('Ctrl Pts',(-4.25131536283724,1.35364300044576,-0.6464684525026));
#18024=CARTESIAN_POINT('Ctrl Pts',(-4.17264475727496,1.28427802017003,0.775177914829204));
#18025=CARTESIAN_POINT('Ctrl Pts',(-4.09397415171266,0.0586940530134323,
1.49894157353371));
#18026=CARTESIAN_POINT('Ctrl Pts',(-4.01530354615037,-1.21973141532996,
0.873227408648153));
#18027=CARTESIAN_POINT('Ctrl Pts',(-3.93663294058809,-1.40004837508882,
-0.538642163332144));
#18028=CARTESIAN_POINT('Ctrl Pts',(-3.85796233502579,-0.319919786174487,
-1.46557912209308));
#18029=CARTESIAN_POINT('Ctrl Pts',(-3.7792917294635,1.04822847243233,-1.07307404333344));
#18030=CARTESIAN_POINT('Ctrl Pts',(-3.70062112390122,1.47267011643486,0.285505797971395));
#18031=CARTESIAN_POINT('Ctrl Pts',(-3.62195051833892,0.571285792138825,
1.38704844050577));
#18032=CARTESIAN_POINT('Ctrl Pts',(-3.54327991277664,-0.844419785166412,
1.239849208655));
#18033=CARTESIAN_POINT('Ctrl Pts',(-3.46460930721434,-1.49990508728209,
-0.0235703231411309));
#18034=CARTESIAN_POINT('Ctrl Pts',(-3.38593870165205,-0.80504512883739,
-1.26576979467919));
#18035=CARTESIAN_POINT('Ctrl Pts',(-3.30726809608976,0.614586610885873,
-1.36841299945646));
#18036=CARTESIAN_POINT('Ctrl Pts',(-3.22859749052747,1.48091392034915,-0.239091572227054));
#18037=CARTESIAN_POINT('Ctrl Pts',(-3.14992688496518,1.01399348485866,1.10548091313801));
#18038=CARTESIAN_POINT('Ctrl Pts',(-3.07125627940289,-0.365812273211845,
1.45480316662115));
#18039=CARTESIAN_POINT('Ctrl Pts',(-2.9925856738406,-1.41628189394276,0.494384801054513));
#18040=CARTESIAN_POINT('Ctrl Pts',(-2.91391506827831,-1.19169123622562,
-0.911121775783751));
#18041=CARTESIAN_POINT('Ctrl Pts',(-2.83524446271602,0.105763904895138,
-1.49635726305551));
#18042=CARTESIAN_POINT('Ctrl Pts',(-2.75657385715373,1.30800080564492,-0.734441302831623));
#18043=CARTESIAN_POINT('Ctrl Pts',(-2.67790325159144,1.33266207978949,0.688682251125587));
#18044=CARTESIAN_POINT('Ctrl Pts',(-2.59923264602915,0.157543528311028,
1.49179491877324));
#18045=CARTESIAN_POINT('Ctrl Pts',(-2.52056204046686,-1.1594069772506,0.951862113425152));
#18046=CARTESIAN_POINT('Ctrl Pts',(-2.44189143490457,-1.4325629685203,-0.445016695197221));
#18047=CARTESIAN_POINT('Ctrl Pts',(-2.36322082934228,-0.415992038324998,
-1.44125881785935));
#18048=CARTESIAN_POINT('Ctrl Pts',(-2.28455022377999,0.975074234532735,
-1.13994251029895));
#18049=CARTESIAN_POINT('Ctrl Pts',(-2.2058796182177,1.48832594768391,0.187627212456071));
#18050=CARTESIAN_POINT('Ctrl Pts',(-2.12720901265541,0.661595609057591,
1.346320752155));
#18051=CARTESIAN_POINT('Ctrl Pts',(-2.04853840709312,-0.76064402464679,
1.29285875853686));
#18052=CARTESIAN_POINT('Ctrl Pts',(-1.96986780153083,-1.49830775742317,
0.0756054196910335));
#18053=CARTESIAN_POINT('Ctrl Pts',(-1.89119719596854,-0.886641406039676,
-1.21000539106371));
#18054=CARTESIAN_POINT('Ctrl Pts',(-1.81252659040624,0.522450526078063,
-1.40570882038797));
#18055=CARTESIAN_POINT('Ctrl Pts',(-1.73385598484396,1.46273493300092,-0.336940454006583));
#18056=CARTESIAN_POINT('Ctrl Pts',(-1.65518537928166,1.08307425741613,1.03732231222955));
#18057=CARTESIAN_POINT('Ctrl Pts',(-1.60273830890681,0.184464955640538,
1.32758424865397));
#18058=CARTESIAN_POINT('Ctrl Pts',(-1.57651477371938,-0.228235294347447,
1.25237280807838));
#18059=CARTESIAN_POINT('Ctrl Pts',(-7.7365,0.684664424539464,-0.958295198918394));
#18060=CARTESIAN_POINT('Ctrl Pts',(-7.71027646481257,1.00045590899587,-0.732674539205356));
#18061=CARTESIAN_POINT('Ctrl Pts',(-7.65782939443771,1.38654401896136,0.0510548484666211));
#18062=CARTESIAN_POINT('Ctrl Pts',(-7.57915878887542,0.718476098825324,
1.1884261498247));
#18063=CARTESIAN_POINT('Ctrl Pts',(-7.50048818331313,-0.596971468671329,
1.25245241149886));
#18064=CARTESIAN_POINT('Ctrl Pts',(-7.42181757775084,-1.37468658999435,
0.190628963548152));
#18065=CARTESIAN_POINT('Ctrl Pts',(-7.34314697218855,-0.914939795064915,
-1.04370829055584));
#18066=CARTESIAN_POINT('Ctrl Pts',(-7.26447636662626,0.368594759353147,
-1.33794018873242));
#18067=CARTESIAN_POINT('Ctrl Pts',(-7.18580576106397,1.32024655518524,-0.427887663681729));
#18068=CARTESIAN_POINT('Ctrl Pts',(-7.10713515550168,1.0833192355362,0.867515846081762));
#18069=CARTESIAN_POINT('Ctrl Pts',(-7.02846454993939,-0.128917960242522,
1.38183808732227));
#18070=CARTESIAN_POINT('Ctrl Pts',(-6.94979394437709,-1.22508593128128,
0.652144954462008));
#18071=CARTESIAN_POINT('Ctrl Pts',(-6.87112333881481,-1.21832796756972,
-0.664684648958273));
#18072=CARTESIAN_POINT('Ctrl Pts',(-6.79245273325251,-0.114723332390545,
-1.38309735453967));
#18073=CARTESIAN_POINT('Ctrl Pts',(-6.71378212769023,1.09216436667117,-0.856330476563782));
#18074=CARTESIAN_POINT('Ctrl Pts',(-6.63511152212794,1.31579099157645,0.441382439659493));
#18075=CARTESIAN_POINT('Ctrl Pts',(-6.55644091656565,0.354827664455788,
1.34172299085838));
#18076=CARTESIAN_POINT('Ctrl Pts',(-6.47777031100335,-0.92558231892019,
1.0341283384462));
#18077=CARTESIAN_POINT('Ctrl Pts',(-6.39909970544107,-1.37270250962841,
-0.204479154130645));
#18078=CARTESIAN_POINT('Ctrl Pts',(-6.32042909987877,-0.583996247497372,
-1.25899648606665));
#18079=CARTESIAN_POINT('Ctrl Pts',(-6.24175849431649,0.73047430811023,-1.18005558026704));
#18080=CARTESIAN_POINT('Ctrl Pts',(-6.1630878887542,1.38730824708363,-0.0387257526847742));
#18081=CARTESIAN_POINT('Ctrl Pts',(-6.0844172831919,0.795166405654621,1.1374683419316));
#18082=CARTESIAN_POINT('Ctrl Pts',(-6.00574667762961,-0.512853522972119,
1.28961433097063));
#18083=CARTESIAN_POINT('Ctrl Pts',(-5.92707607206732,-1.35915802111573,
0.280737112808016));
#18084=CARTESIAN_POINT('Ctrl Pts',(-5.84840546650503,-0.981830029670403,
-0.980884113613565));
#18085=CARTESIAN_POINT('Ctrl Pts',(-5.76973486094274,0.279426911638065,
-1.3594279881432));
#18086=CARTESIAN_POINT('Ctrl Pts',(-5.69106425538045,1.28911939778457,-0.514096324773416));
#18087=CARTESIAN_POINT('Ctrl Pts',(-5.61239364981816,1.13823426692583,0.794069648334226));
#18088=CARTESIAN_POINT('Ctrl Pts',(-5.53372304425587,-0.0373885377105224,
1.38734492840875));
#18089=CARTESIAN_POINT('Ctrl Pts',(-5.45505243869358,-1.17935092265908,
0.731611409282145));
#18090=CARTESIAN_POINT('Ctrl Pts',(-5.37638183313129,-1.25955883732489,
-0.582782453657743));
#18091=CARTESIAN_POINT('Ctrl Pts',(-5.297711227569,-0.205802127560476,-1.37250476768144));
#18092=CARTESIAN_POINT('Ctrl Pts',(-5.21904062200671,1.03323559121881,-0.926578688525379));
#18093=CARTESIAN_POINT('Ctrl Pts',(-5.14037001644442,1.34206459371129,0.353534268919763));
#18094=CARTESIAN_POINT('Ctrl Pts',(-5.06169941088212,0.442650100242435,
1.31536487019939));
#18095=CARTESIAN_POINT('Ctrl Pts',(-4.98302880531984,-0.855276586389133,
1.0929893932559));
#18096=CARTESIAN_POINT('Ctrl Pts',(-4.90435819975755,-1.38320876038964,
-0.113390379563494));
#18097=CARTESIAN_POINT('Ctrl Pts',(-4.82568759419526,-0.66585587424462,
-1.21768625176223));
#18098=CARTESIAN_POINT('Ctrl Pts',(-4.74701698863296,0.650958493169218,
-1.22571484985989));
#18099=CARTESIAN_POINT('Ctrl Pts',(-4.66834638307068,1.38172329992943,-0.130248130230639));
#18100=CARTESIAN_POINT('Ctrl Pts',(-4.58967577750838,0.868540387494536,
1.08247930617046));
#18101=CARTESIAN_POINT('Ctrl Pts',(-4.5110051719461,-0.42657826714551,1.32066454294621));
#18102=CARTESIAN_POINT('Ctrl Pts',(-4.4323345663838,-1.33765399329139,0.36987247427784));
#18103=CARTESIAN_POINT('Ctrl Pts',(-4.35366396082152,-1.04445703031594,
-0.913911026752496));
#18104=CARTESIAN_POINT('Ctrl Pts',(-4.27499335525923,0.189051166264626,
-1.37491218247906));
#18105=CARTESIAN_POINT('Ctrl Pts',(-4.19632274969693,1.25235902888845,-0.598097580467343));
#18106=CARTESIAN_POINT('Ctrl Pts',(-4.11765214413465,1.18818416202297,0.717176582238888));
#18107=CARTESIAN_POINT('Ctrl Pts',(-4.03898153857235,0.0543023730844936,
1.38678589020371));
#18108=CARTESIAN_POINT('Ctrl Pts',(-3.96031093301006,-1.12846714407295,
0.807889694057623));
#18109=CARTESIAN_POINT('Ctrl Pts',(-3.88164032744778,-1.295292202483,-0.498339204921006));
#18110=CARTESIAN_POINT('Ctrl Pts',(-3.80296972188548,-0.295982347342492,
-1.35591972587991));
#18111=CARTESIAN_POINT('Ctrl Pts',(-3.72429911632319,0.969796609117977,
-0.992783153602477));
#18112=CARTESIAN_POINT('Ctrl Pts',(-3.6456285107609,1.36248014896398,0.264143325656574));
#18113=CARTESIAN_POINT('Ctrl Pts',(-3.56695790519861,0.528540331258045,
1.28326496528333));
#18114=CARTESIAN_POINT('Ctrl Pts',(-3.48828729963633,-0.781237550651807,
1.14707965867511));
#18115=CARTESIAN_POINT('Ctrl Pts',(-3.40961669407403,-1.38767731071994,
-0.0218067149092513));
#18116=CARTESIAN_POINT('Ctrl Pts',(-3.33094608851175,-0.744809034162001,
-1.17106078215508));
#18117=CARTESIAN_POINT('Ctrl Pts',(-3.25227548294945,0.568601241925253,
-1.26602388853876));
#18118=CARTESIAN_POINT('Ctrl Pts',(-3.17360487738716,1.37010712465924,-0.22120196322891));
#18119=CARTESIAN_POINT('Ctrl Pts',(-3.09493427182487,0.938123194652226,
1.02276523601594));
#18120=CARTESIAN_POINT('Ctrl Pts',(-3.01626366626258,-0.338441009250009,
1.34595006244152));
#18121=CARTESIAN_POINT('Ctrl Pts',(-2.93759306070029,-1.31031107666228,
0.457393322421008));
#18122=CARTESIAN_POINT('Ctrl Pts',(-2.858922455138,-1.10252502236034,-0.842948681405594));
#18123=CARTESIAN_POINT('Ctrl Pts',(-2.78025184957571,0.0978503055697247,
-1.38439494624008));
#18124=CARTESIAN_POINT('Ctrl Pts',(-2.70158124401342,1.21013193153834,-0.679488016032942));
#18125=CARTESIAN_POINT('Ctrl Pts',(-2.62291063845113,1.232947968949,0.637152805391334));
#18126=CARTESIAN_POINT('Ctrl Pts',(-2.54424003288884,0.145755609165987,
1.38017397139449));
#18127=CARTESIAN_POINT('Ctrl Pts',(-2.46556942732655,-1.07265637663543,
0.880640694490544));
#18128=CARTESIAN_POINT('Ctrl Pts',(-2.38689882176426,-1.32537394829127,
-0.411719098796964));
#18129=CARTESIAN_POINT('Ctrl Pts',(-2.30822821620197,-0.384866161144742,
-1.33341914590248));
#18130=CARTESIAN_POINT('Ctrl Pts',(-2.22955761063968,0.902116009207335,
-1.05464830440266));
#18131=CARTESIAN_POINT('Ctrl Pts',(-2.15088700507739,1.37696456000371,0.173588334226353));
#18132=CARTESIAN_POINT('Ctrl Pts',(-2.0722163995151,0.612092873972952,1.24558465502793));
#18133=CARTESIAN_POINT('Ctrl Pts',(-1.9935457939528,-0.703730164986462,
1.19612286163926));
#18134=CARTESIAN_POINT('Ctrl Pts',(-1.91487518839052,-1.38619949827584,
0.069948376308802));
#18135=CARTESIAN_POINT('Ctrl Pts',(-1.83620458282822,-0.820300012539843,
-1.11946885257289));
#18136=CARTESIAN_POINT('Ctrl Pts',(-1.75753397726593,0.483359078624077,
-1.30052911485619));
#18137=CARTESIAN_POINT('Ctrl Pts',(-1.67886337170364,1.35328834826538,-0.31172947345345));
#18138=CARTESIAN_POINT('Ctrl Pts',(-1.60019276614135,1.0020351191452,0.959706483290145));
#18139=CARTESIAN_POINT('Ctrl Pts',(-1.54774569576649,0.170662687749908,
1.22825007765296));
#18140=CARTESIAN_POINT('Ctrl Pts',(-1.52152216057906,-0.211157987366626,
1.15866620166089));
#18141=CARTESIAN_POINT('Ctrl Pts',(-1.6865,-0.262389908309069,1.43978602091337));
#18142=CARTESIAN_POINT('Ctrl Pts',(-1.71272353518743,0.212069491421808,
1.52625259065599));
#18143=CARTESIAN_POINT('Ctrl Pts',(-1.73894707037486,0.728611012689902,
1.35940328038217));
#18144=CARTESIAN_POINT('Ctrl Pts',(-1.76517060556229,1.05962770140961,1.01265922770839));
#18145=CARTESIAN_POINT('Ctrl Pts',(-1.79139414074972,1.39064439012933,0.665915175034609));
#18146=CARTESIAN_POINT('Ctrl Pts',(-1.81761767593715,1.53613624630066,0.139276379960869));
#18147=CARTESIAN_POINT('Ctrl Pts',(-1.84384121112458,1.42871639413866,-0.328827320299109));
#18148=CARTESIAN_POINT('Ctrl Pts',(-1.87006474631201,1.32129654197666,-0.796931020559087));
#18149=CARTESIAN_POINT('Ctrl Pts',(-1.89628828149944,0.960964981481353,
-1.2064996260053));
#18150=CARTESIAN_POINT('Ctrl Pts',(-1.92251181668687,0.510806265562799,
-1.37378563482738));
#18151=CARTESIAN_POINT('Ctrl Pts',(-1.9487353518743,0.0606475496442437,
-1.54107164364947));
#18152=CARTESIAN_POINT('Ctrl Pts',(-1.97495888706173,-0.479338321697556,
-1.46607505584741));
#18153=CARTESIAN_POINT('Ctrl Pts',(-2.00118242224916,-0.866531271148201,
-1.18224376619624));
#18154=CARTESIAN_POINT('Ctrl Pts',(-2.02606993288514,-1.23399769315247,
-0.912872981916841));
#18155=CARTESIAN_POINT('Ctrl Pts',(-2.05095744352111,-1.46384344241319,
-0.455404661410297));
#18156=CARTESIAN_POINT('Ctrl Pts',(-2.07584495415709,-1.46567283994288,
0.000450589203851749));
#18157=CARTESIAN_POINT('Origin',(-1.69543030951378,0.,0.));
#18158=CARTESIAN_POINT('',(-2.00086061902756,0.,0.));
#18159=CARTESIAN_POINT('',(-1.4,-0.983629653494575,1.20459890669855E-16));
#18160=CARTESIAN_POINT('',(-1.69543030951378,-0.5,-6.12323399573677E-17));
#18161=CARTESIAN_POINT('Origin',(-1.4,0.,0.));
#18162=CARTESIAN_POINT('Origin',(0.,1.38777878078145E-16,1.15470053837925));
#18163=CARTESIAN_POINT('',(0.,7.07050159149938E-17,1.15470053837925));
#18164=CARTESIAN_POINT('',(0.,1.,0.577350269189626));
#18165=CARTESIAN_POINT('',(0.,0.25,1.01036297108185));
#18166=CARTESIAN_POINT('',(-1.4,1.38777878078145E-16,1.15470053837925));
#18167=CARTESIAN_POINT('',(0.,7.07050159149938E-17,1.15470053837925));
#18168=CARTESIAN_POINT('',(-1.4,1.,0.577350269189626));
#18169=CARTESIAN_POINT('',(-1.4,1.,0.577350269189626));
#18170=CARTESIAN_POINT('',(0.,1.,0.577350269189626));
#18171=CARTESIAN_POINT('Origin',(0.,-1.,0.577350269189626));
#18172=CARTESIAN_POINT('',(0.,-1.,0.577350269189626));
#18173=CARTESIAN_POINT('',(0.,-0.75,0.721687836487032));
#18174=CARTESIAN_POINT('',(-1.4,-1.,0.577350269189626));
#18175=CARTESIAN_POINT('',(0.,-1.,0.577350269189626));
#18176=CARTESIAN_POINT('',(-1.4,7.07050159149938E-17,1.15470053837925));
#18177=CARTESIAN_POINT('Origin',(0.,-1.,-0.577350269189626));
#18178=CARTESIAN_POINT('',(0.,-1.,-0.577350269189626));
#18179=CARTESIAN_POINT('',(0.,-1.,-0.288675134594813));
#18180=CARTESIAN_POINT('',(-1.4,-1.,-0.577350269189626));
#18181=CARTESIAN_POINT('',(0.,-1.,-0.577350269189626));
#18182=CARTESIAN_POINT('',(-1.4,-1.,0.577350269189626));
#18183=CARTESIAN_POINT('Origin',(0.,-2.77555756156289E-16,-1.15470053837925));
#18184=CARTESIAN_POINT('',(0.,-2.12115047744981E-16,-1.15470053837925));
#18185=CARTESIAN_POINT('',(0.,-0.25,-1.01036297108185));
#18186=CARTESIAN_POINT('',(-1.4,-2.77555756156289E-16,-1.15470053837925));
#18187=CARTESIAN_POINT('',(0.,-2.12115047744981E-16,-1.15470053837925));
#18188=CARTESIAN_POINT('',(-1.4,-1.,-0.577350269189626));
#18189=CARTESIAN_POINT('Origin',(0.,1.,-0.577350269189626));
#18190=CARTESIAN_POINT('',(0.,1.,-0.577350269189626));
#18191=CARTESIAN_POINT('',(0.,0.75,-0.721687836487033));
#18192=CARTESIAN_POINT('',(-1.4,1.,-0.577350269189626));
#18193=CARTESIAN_POINT('',(0.,1.,-0.577350269189626));
#18194=CARTESIAN_POINT('',(-1.4,-2.12115047744981E-16,-1.15470053837925));
#18195=CARTESIAN_POINT('Origin',(0.,1.,0.577350269189626));
#18196=CARTESIAN_POINT('',(0.,1.,0.288675134594813));
#18197=CARTESIAN_POINT('',(-1.4,1.,-0.577350269189626));
#18198=CARTESIAN_POINT('Origin',(-1.4,0.,0.));
#18199=CARTESIAN_POINT('Origin',(-8.,1.2,0.));
#18200=CARTESIAN_POINT('',(-8.,-1.2,-1.46957615897682E-16));
#18201=CARTESIAN_POINT('Origin',(-8.,0.,0.));
#18202=CARTESIAN_POINT('Origin',(-7.85,0.,0.));
#18203=CARTESIAN_POINT('',(-7.85,-1.35,-1.65327317884893E-16));
#18204=CARTESIAN_POINT('Origin',(-4.675,0.,0.));
#18205=CARTESIAN_POINT('Origin',(-1.6865,0.,0.));
#18206=CARTESIAN_POINT('Origin',(-0.825,0.,0.));
#18207=CARTESIAN_POINT('',(0.,-3.15,-3.85763741731416E-16));
#18208=CARTESIAN_POINT('Origin',(0.,0.,0.));
#18209=CARTESIAN_POINT('',(-0.825,-2.325,-2.8473038080176E-16));
#18210=CARTESIAN_POINT('Origin',(0.,0.,0.));
#18264=UNCERTAINTY_MEASURE_WITH_UNIT(LENGTH_MEASURE(0.01),#18282,
'DISTANCE_ACCURACY_VALUE',
'Maximum model space distance between geometric entities at asserted c
onnectivities');
#18266=UNCERTAINTY_MEASURE_WITH_UNIT(LENGTH_MEASURE(0.01),#18282,
'DISTANCE_ACCURACY_VALUE',
'Maximum model space distance between geometric entities at asserted c
onnectivities');
#18279=(
GEOMETRIC_REPRESENTATION_CONTEXT(3)
GLOBAL_UNCERTAINTY_ASSIGNED_CONTEXT((#18264))
GLOBAL_UNIT_ASSIGNED_CONTEXT((#18282,#18284,#18285))
REPRESENTATION_CONTEXT('','3D')
);
#18281=(
GEOMETRIC_REPRESENTATION_CONTEXT(3)
GLOBAL_UNCERTAINTY_ASSIGNED_CONTEXT((#18266))
GLOBAL_UNIT_ASSIGNED_CONTEXT((#18282,#18284,#18285))
REPRESENTATION_CONTEXT('','3D')
);
#18282=(
LENGTH_UNIT()
NAMED_UNIT(*)
SI_UNIT(.MILLI.,.METRE.)
);
#18284=(
NAMED_UNIT(*)
PLANE_ANGLE_UNIT()
SI_UNIT($,.RADIAN.)
);
#18285=(
NAMED_UNIT(*)
SI_UNIT($,.STERADIAN.)
SOLID_ANGLE_UNIT()
);
#18298=SHAPE_DEFINITION_REPRESENTATION(#18312,#18350);
#18312=PRODUCT_DEFINITION_SHAPE('',$,#18365);
#18350=SHAPE_REPRESENTATION('',(#9884),#18279);
#18352=PRODUCT_DEFINITION_CONTEXT('part definition',#18396,'design');
#18365=PRODUCT_DEFINITION('2026-10-20-13-03-25-859','11_ISO_10642_M3x8',
#18379,#18352);
#18379=PRODUCT_DEFINITION_FORMATION('',$,#18410);
#18396=APPLICATION_CONTEXT(
'Core Data for Automotive Mechanical Design Process');
#18397=PRODUCT_CONTEXT('part definition',#18396,'mechanical');
#18410=PRODUCT('2026-10-20-13-03-25-859','11_ISO_10642_M3x8',$,(#18397));
#18475=COLOUR_RGB('Black',0.12,0.14,0.17);
#18476=FILL_AREA_STYLE_COLOUR('',#18475);
#18477=FILL_AREA_STYLE('',(#18476));
#18478=SURFACE_STYLE_FILL_AREA(#18477);
#18479=SURFACE_SIDE_STYLE('',(#18478));
#18480=SURFACE_STYLE_USAGE(.BOTH.,#18479);
#18481=PRESENTATION_STYLE_ASSIGNMENT((#18480));
ENDSEC;
END-ISO-10303-21;
